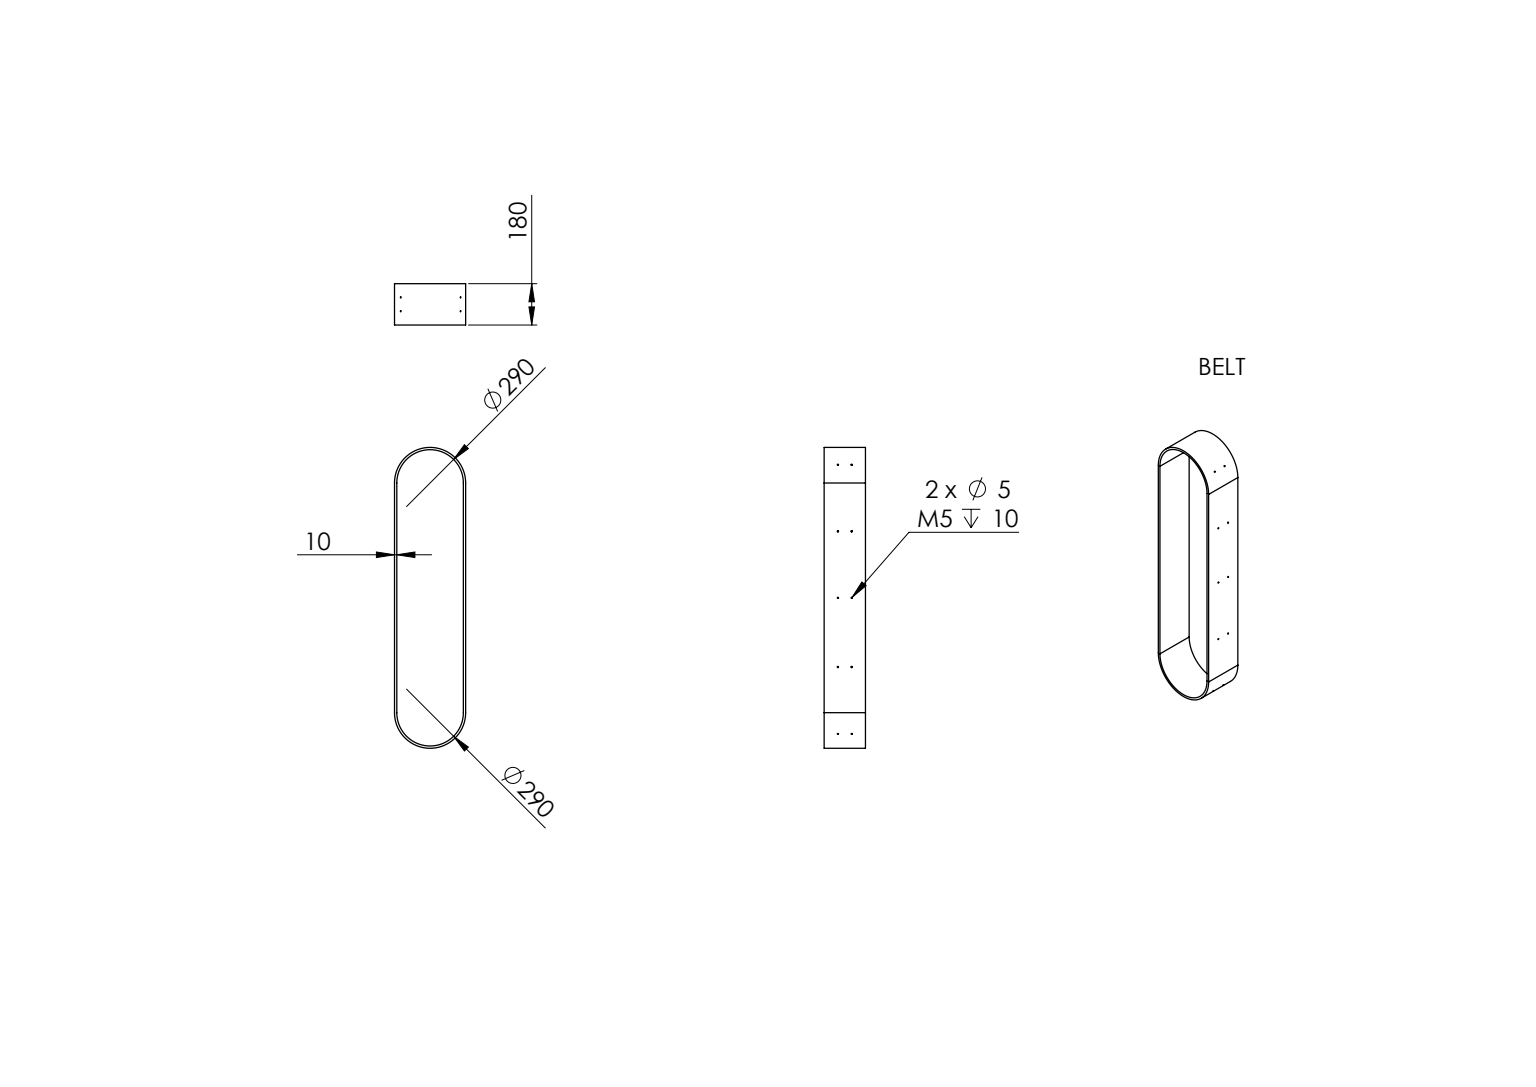
ISO-10303-21;
HEADER;
FILE_DESCRIPTION (('STEP AP214'),
    '1' );
FILE_NAME ('belt.step',
    '2026-10-31T03:46:07',
    ( '' ),
    ( '' ),
    'SwSTEP 2.0',
    'SolidWorks 2026',
    '' );
FILE_SCHEMA (( 'AUTOMOTIVE_DESIGN' ));
ENDSEC;

DATA;
#1=DIRECTION ( 'NONE',  ( -0.000000000000000000, -0.000000000000000000, -1.000000000000000000 ) ) ;
#9=CARTESIAN_POINT ( 'NONE',  ( 155.0000000000000568, -1000.000000000000000, 90.00000000000000000 ) ) ;
#15=AXIS2_PLACEMENT_3D ( 'NONE', #6057, #12994, #3756 ) ;
#18=CIRCLE ( 'NONE', #21621, 2.499999999999998668 ) ;
#25=CARTESIAN_POINT ( 'NONE',  ( -128.2695163047654319, 87.01699568756248482, -27.57873596473009670 ) ) ;
#36=CARTESIAN_POINT ( 'NONE',  ( -146.0000000000001137, -204.4690652294807478, 27.94500000000641649 ) ) ;
#37=LINE ( 'NONE', #254, #11884 ) ;
#45=VERTEX_POINT ( 'NONE', #9 ) ;
#55=DIRECTION ( 'NONE',  ( 0.9289202219288174023, 0.3702799228849934510, 6.982962677686266711E-15 ) ) ;
#56=CARTESIAN_POINT ( 'NONE',  ( 133.4872637682705090, 78.77924338079024835, 32.17229779615544771 ) ) ;
#74=CARTESIAN_POINT ( 'NONE',  ( 126.3653543294811499, 77.28387428943223370, 30.00000000000641620 ) ) ;
#82=LINE ( 'NONE', #14822, #8863 ) ;
#83=FACE_OUTER_BOUND ( 'NONE', #5048, .T. ) ;
#104=DIRECTION ( 'NONE',  ( 0.4924295582441756136, -0.5074575156280946020, -0.7071067811865532349 ) ) ;
#107=EDGE_CURVE ( 'NONE', #20023, #9785, #19883, .T. ) ;
#111=CARTESIAN_POINT ( 'NONE',  ( -127.8094121079449081, 87.69139705313254751, -27.49999999999350919 ) ) ;
#113=CYLINDRICAL_SURFACE ( 'NONE', #13258, 2.500000000000002220 ) ;
#120=LINE ( 'NONE', #7470, #18771 ) ;
#144=CARTESIAN_POINT ( 'NONE',  ( -136.7455495141632014, -1072.977142426286946, -31.53250949154617189 ) ) ;
#149=EDGE_CURVE ( 'NONE', #7198, #16229, #4462, .T. ) ;
#150=CARTESIAN_POINT ( 'NONE',  ( -134.5566256099404825, -1076.938388239963842, 30.33200430454444785 ) ) ;
#153=ADVANCED_FACE ( 'NONE', ( #23660 ), #11773, .F. ) ;
#159=CARTESIAN_POINT ( 'NONE',  ( 125.5946212300931251, -1090.835042168281007, 31.66065886938999796 ) ) ;
#161=CARTESIAN_POINT ( 'NONE',  ( -129.3084827928275899, 85.46529914716332144, 30.33200430454444785 ) ) ;
#166=FACE_OUTER_BOUND ( 'NONE', #524, .T. ) ;
#170=B_SPLINE_CURVE_WITH_KNOTS ( 'NONE', 3,
 ( #22399, #16491, #3559, #1745, #10973, #23729, #1990, #12913, #5622, #7185, #14575, #13162, #16380, #9267, #21916, #7319, #18537, #13033, #1867, #10867, #14821, #16628, #20334, #18294, #9136, #12812, #18638, #15068, #11086, #11248, #14938, #14705 ),
 .UNSPECIFIED., .F., .F.,
 ( 4, 2, 2, 2, 2, 2, 2, 2, 2, 2, 2, 2, 2, 2, 2, 4 ),
 ( 1.551583845779545699E-17, 0.0004914281572964048763, 0.0009828563145927943570, 0.001474284471889183512, 0.001965712629185573102, 0.002457140786481962474, 0.002948568943778351412, 0.003931425258371110641, 0.004422853415667485702, 0.004914281572963859895, 0.005405709730260234956, 0.005897137887556608282, 0.006388566044852983343, 0.006879994202149357536, 0.007371422359445732597, 0.007862850516742106791 ),
 .UNSPECIFIED. ) ;
#173=CARTESIAN_POINT ( 'NONE',  ( 131.5154891841473841, 82.02850787876496952, -30.32849798811265885 ) ) ;
#178=AXIS2_PLACEMENT_3D ( 'NONE', #20566, #18993, #2455 ) ;
#181=AXIS2_PLACEMENT_3D ( 'NONE', #11379, #9543, #20890 ) ;
#184=DIRECTION ( 'NONE',  ( 0.000000000000000000, -1.000000000000000000, 0.000000000000000000 ) ) ;
#189=DIRECTION ( 'NONE',  ( 0.9289202219288174023, 0.3702799228849934510, 6.982962677686266711E-15 ) ) ;
#190=ORIENTED_EDGE ( 'NONE', *, *, #703, .F. ) ;
#192=DIRECTION ( 'NONE',  ( -0.9289202219288174023, -0.3702799228849933955, -6.982962677686267499E-15 ) ) ;
#204=CARTESIAN_POINT ( 'NONE',  ( 194.7499999999997442, -209.9999999999996874, 30.00000000000675726 ) ) ;
#208=DIRECTION ( 'NONE',  ( -1.350636282998972974E-14, 0.000000000000000000, -1.000000000000000000 ) ) ;
#221=CARTESIAN_POINT ( 'NONE',  ( -135.9481979339306577, -1074.452087582500553, 27.51597717546056643 ) ) ;
#223=VERTEX_POINT ( 'NONE', #18684 ) ;
#242=ORIENTED_EDGE ( 'NONE', *, *, #6175, .T. ) ;
#250=DIRECTION ( 'NONE',  ( -0.000000000000000000, -0.000000000000000000, -1.000000000000000000 ) ) ;
#254=CARTESIAN_POINT ( 'NONE',  ( 194.7500000000001705, -210.0000000000003411, -27.49999999999322498 ) ) ;
#274=ORIENTED_EDGE ( 'NONE', *, *, #4252, .F. ) ;
#275=CARTESIAN_POINT ( 'NONE',  ( 125.1337793500219817, -1091.468903702553689, 27.75096515221187232 ) ) ;
#277=AXIS2_PLACEMENT_3D ( 'NONE', #7099, #10883, #12700 ) ;
#278=CARTESIAN_POINT ( 'NONE',  ( -127.9949300873395543, 87.42039156790949050, 32.50000000000647304 ) ) ;
#279=EDGE_CURVE ( 'NONE', #7198, #16055, #16896, .T. ) ;
#283=ORIENTED_EDGE ( 'NONE', *, *, #21682, .F. ) ;
#288=EDGE_CURVE ( 'NONE', #16653, #6623, #20746, .T. ) ;
#290=CARTESIAN_POINT ( 'NONE',  ( 132.6714475832646656, 80.14557597090949059, -27.51562286569268423 ) ) ;
#295=VECTOR ( 'NONE', #20136, 1000.000000000000000 ) ;
#299=ORIENTED_EDGE ( 'NONE', *, *, #12045, .F. ) ;
#314=AXIS2_PLACEMENT_3D ( 'NONE', #11031, #20164, #12506 ) ;
#323=CYLINDRICAL_SURFACE ( 'NONE', #9568, 2.500000000000002220 ) ;
#349=ORIENTED_EDGE ( 'NONE', *, *, #18259, .F. ) ;
#360=AXIS2_PLACEMENT_3D ( 'NONE', #12995, #16243, #18159 ) ;
#361=CIRCLE ( 'NONE', #6148, 2.055000000000001492 ) ;
#365=CARTESIAN_POINT ( 'NONE',  ( -127.2680799365782889, 88.47518962644093676, 27.75040112528346015 ) ) ;
#371=AXIS2_PLACEMENT_3D ( 'NONE', #23355, #14098, #23119 ) ;
#378=EDGE_LOOP ( 'NONE', ( #19734, #5802 ) ) ;
#380=VECTOR ( 'NONE', #18750, 1000.000000000000114 ) ;
#392=ORIENTED_EDGE ( 'NONE', *, *, #11920, .F. ) ;
#394=AXIS2_PLACEMENT_3D ( 'NONE', #13322, #2647, #11500 ) ;
#401=CARTESIAN_POINT ( 'NONE',  ( -135.6291186032800340, -1075.032345129804526, 27.50000000000644462 ) ) ;
#404=VERTEX_POINT ( 'NONE', #6272 ) ;
#412=CARTESIAN_POINT ( 'NONE',  ( -128.8385278530645905, 86.17219694792730422, 28.11255663403418126 ) ) ;
#415=EDGE_CURVE ( 'NONE', #12774, #3203, #17606, .T. ) ;
#420=ORIENTED_EDGE ( 'NONE', *, *, #2725, .F. ) ;
#426=CARTESIAN_POINT ( 'NONE',  ( 132.5032837044622056, 80.42329363488276783, -27.57873596473011446 ) ) ;
#439=DIRECTION ( 'NONE',  ( 1.000000000000000000, -0.000000000000000000, 6.982962677686266711E-15 ) ) ;
#455=ORIENTED_EDGE ( 'NONE', *, *, #19160, .F. ) ;
#457=CARTESIAN_POINT ( 'NONE',  ( 153.5653415408403646, -1122.352966361445169, 30.00000000000675726 ) ) ;
#462=DIRECTION ( 'NONE',  ( -0.7232617928448825673, 0.6905739489807055653, 6.982962677686266711E-15 ) ) ;
#471=VERTEX_POINT ( 'NONE', #10993 ) ;
#480=CARTESIAN_POINT ( 'NONE',  ( -146.4450000000005332, -784.4690652294799520, -29.99999999999356248 ) ) ;
#483=CARTESIAN_POINT ( 'NONE',  ( -127.9021285790841205, 87.55595642181887683, 27.50000000000646239 ) ) ;
#493=VERTEX_POINT ( 'NONE', #1420 ) ;
#507=CARTESIAN_POINT ( 'NONE',  ( -136.9304241666588666, -1072.629629052829387, -29.19154146838981490 ) ) ;
#512=ORIENTED_EDGE ( 'NONE', *, *, #2203, .T. ) ;
#513=DIRECTION ( 'NONE',  ( -0.7071067811865320296, 9.875400524328840493E-15, 0.7071067811865631159 ) ) ;
#524=EDGE_LOOP ( 'NONE', ( #4189, #16667, #22630, #21113 ) ) ;
#547=ORIENTED_EDGE ( 'NONE', *, *, #19326, .F. ) ;
#572=ORIENTED_EDGE ( 'NONE', *, *, #16103, .T. ) ;
#586=CARTESIAN_POINT ( 'NONE',  ( -146.0000000000005684, -496.5240652294801293, -29.99999999999356604 ) ) ;
#590=VERTEX_POINT ( 'NONE', #22650 ) ;
#597=DIRECTION ( 'NONE',  ( 1.000000000000000000, -0.000000000000000000, 6.982962677686266711E-15 ) ) ;
#598=CARTESIAN_POINT ( 'NONE',  ( -126.4561707720357191, 89.63167338449062527, 29.67072815018523357 ) ) ;
#619=EDGE_CURVE ( 'NONE', #20328, #13113, #6356, .T. ) ;
#624=CARTESIAN_POINT ( 'NONE',  ( -136.9597779064870053, -1072.574344195403910, -30.66034227022094072 ) ) ;
#634=DIRECTION ( 'NONE',  ( -1.000000000000000000, 1.408839003528726857E-14, 6.982962677686266711E-15 ) ) ;
#648=CARTESIAN_POINT ( 'NONE',  ( 155.0000000000000568, -801.0618695410399823, 32.50000000000648015 ) ) ;
#656=DIRECTION ( 'NONE',  ( 1.350636282998972974E-14, 0.000000000000000000, -1.000000000000000000 ) ) ;
#658=ORIENTED_EDGE ( 'NONE', *, *, #12364, .F. ) ;
#667=VECTOR ( 'NONE', #14846, 1000.000000000000114 ) ;
#676=VECTOR ( 'NONE', #16342, 1000.000000000000000 ) ;
#677=DIRECTION ( 'NONE',  ( 1.350636282998972974E-14, 0.000000000000000000, -1.000000000000000000 ) ) ;
#703=EDGE_CURVE ( 'NONE', #23044, #590, #11400, .T. ) ;
#706=EDGE_CURVE ( 'NONE', #3521, #2188, #19499, .T. ) ;
#716=ORIENTED_EDGE ( 'NONE', *, *, #17409, .T. ) ;
#717=ORIENTED_EDGE ( 'NONE', *, *, #4723, .F. ) ;
#726=DIRECTION ( 'NONE',  ( 1.000000000000000000, -0.000000000000000000, 6.982962677686266711E-15 ) ) ;
#732=DIRECTION ( 'NONE',  ( -0.000000000000000000, 0.000000000000000000, -1.000000000000000000 ) ) ;
#742=ADVANCED_FACE ( 'NONE', ( #13655 ), #12191, .F. ) ;
#750=CARTESIAN_POINT ( 'NONE',  ( -127.9021285790841205, 87.55595642181886262, 32.50000000000646594 ) ) ;
#782=CIRCLE ( 'NONE', #20051, 2.499999999999998668 ) ;
#784=VERTEX_POINT ( 'NONE', #15907 ) ;
#790=EDGE_CURVE ( 'NONE', #2904, #12317, #6354, .T. ) ;
#794=CARTESIAN_POINT ( 'NONE',  ( -135.7895026000616951, -1074.740959209979792, -32.49999999999351985 ) ) ;
#800=ORIENTED_EDGE ( 'NONE', *, *, #9748, .T. ) ;
#802=DIRECTION ( 'NONE',  ( -1.350636282998972974E-14, 0.000000000000000000, -1.000000000000000000 ) ) ;
#803=DIRECTION ( 'NONE',  ( 1.110223024625157172E-14, 0.000000000000000000, -1.000000000000000000 ) ) ;
#816=ADVANCED_FACE ( 'NONE', ( #4674 ), #21087, .F. ) ;
#825=EDGE_LOOP ( 'NONE', ( #14289, #18811, #20424, #21702 ) ) ;
#828=DIRECTION ( 'NONE',  ( 0.000000000000000000, 0.000000000000000000, -1.000000000000000000 ) ) ;
#834=CARTESIAN_POINT ( 'NONE',  ( -134.7167544493340472, -1076.657711551589273, -28.73951976925632223 ) ) ;
#846=VERTEX_POINT ( 'NONE', #23494 ) ;
#854=ORIENTED_EDGE ( 'NONE', *, *, #6766, .T. ) ;
#860=ORIENTED_EDGE ( 'NONE', *, *, #4723, .T. ) ;
#871=EDGE_CURVE ( 'NONE', #8499, #16240, #17927, .T. ) ;
#885=VERTEX_POINT ( 'NONE', #4487 ) ;
#886=FACE_OUTER_BOUND ( 'NONE', #15033, .T. ) ;
#900=DIRECTION ( 'NONE',  ( 0.7071067811865320296, 8.659560562355062281E-17, 0.7071067811865631159 ) ) ;
#902=FACE_OUTER_BOUND ( 'NONE', #12806, .T. ) ;
#907=VERTEX_POINT ( 'NONE', #17295 ) ;
#910=CARTESIAN_POINT ( 'NONE',  ( 145.0000000000000284, 0.000000000000000000, -90.00000000000000000 ) ) ;
#911=ADVANCED_FACE ( 'NONE', ( #9367 ), #17415, .F. ) ;
#924=DIRECTION ( 'NONE',  ( -1.000000000000000000, 1.408839003528726857E-14, 6.982962677686266711E-15 ) ) ;
#927=CARTESIAN_POINT ( 'NONE',  ( -146.0000000000000568, -784.4690652294805204, 32.05500000000641592 ) ) ;
#941=CARTESIAN_POINT ( 'NONE',  ( -127.9021285790841205, 87.55595642181886262, 32.50000000000646594 ) ) ;
#942=CIRCLE ( 'NONE', #6346, 2.500000000000002220 ) ;
#944=CARTESIAN_POINT ( 'NONE',  ( -135.2464651929980164, -1075.719328653694674, -32.24903484778816676 ) ) ;
#946=CONICAL_SURFACE ( 'NONE', #22543, 2.055000000000001492, 0.7853981633974633780 ) ;
#950=ORIENTED_EDGE ( 'NONE', *, *, #15583, .F. ) ;
#951=CARTESIAN_POINT ( 'NONE',  ( 133.6256533058505340, 78.54427823740819292, -31.99339931332764664 ) ) ;
#963=VERTEX_POINT ( 'NONE', #1980 ) ;
#970=AXIS2_PLACEMENT_3D ( 'NONE', #14005, #15567, #10496 ) ;
#979=ORIENTED_EDGE ( 'NONE', *, *, #3400, .T. ) ;
#984=EDGE_LOOP ( 'NONE', ( #10266, #7109, #23635, #16321 ) ) ;
#992=CARTESIAN_POINT ( 'NONE',  ( -155.0000000000000284, -784.4690652294804067, 30.00000000000648015 ) ) ;
#998=FACE_OUTER_BOUND ( 'NONE', #17064, .T. ) ;
#1013=DIRECTION ( 'NONE',  ( -0.7232617928448825673, 0.6905739489807055653, 6.982962677686266711E-15 ) ) ;
#1014=ORIENTED_EDGE ( 'NONE', *, *, #14681, .T. ) ;
#1026=CARTESIAN_POINT ( 'NONE',  ( 132.1831532210145781, 80.94878845338391216, 32.18904844917290831 ) ) ;
#1028=EDGE_CURVE ( 'NONE', #3982, #8260, #19323, .T. ) ;
#1034=CARTESIAN_POINT ( 'NONE',  ( 145.9999999999997726, -209.9999999999996874, 32.05500000000641592 ) ) ;
#1052=B_SPLINE_CURVE_WITH_KNOTS ( 'NONE', 3,
 ( #9232, #278, #22370, #3531, #9350, #10941, #2076, #20438, #7635, #13244, #13126, #18510, #14673, #161, #12780, #11057, #16464, #1716, #20548, #1964, #7407, #412, #3999, #11418, #15149, #2190, #14906, #9583 ),
 .UNSPECIFIED., .F., .F.,
 ( 4, 2, 2, 2, 2, 2, 2, 2, 2, 2, 2, 2, 2, 4 ),
 ( 0.007862850516742138016, 0.008354729399060728881, 0.008846608281379319746, 0.009830366046016465048, 0.01032224492833501775, 0.01081412381065357219, 0.01130600269297213530, 0.01179788157529069667, 0.01278163933992781248, 0.01327351822224636518, 0.01376539710456491789, 0.01425727598688347232, 0.01474915486920202502, 0.01573291263383913910 ),
 .UNSPECIFIED. ) ;
#1060=DIRECTION ( 'NONE',  ( 6.982962677686266711E-15, -9.837870180509810443E-29, 1.000000000000000000 ) ) ;
#1066=ORIENTED_EDGE ( 'NONE', *, *, #17131, .T. ) ;
#1070=EDGE_LOOP ( 'NONE', ( #5859, #20179, #7990, #3213 ) ) ;
#1071=CARTESIAN_POINT ( 'NONE',  ( 134.1261853992453723, 77.68633335585815303, -30.32927184981474866 ) ) ;
#1074=EDGE_CURVE ( 'NONE', #19239, #3203, #19111, .T. ) ;
#1078=DIRECTION ( 'NONE',  ( 0.000000000000000000, 0.000000000000000000, -1.000000000000000000 ) ) ;
#1086=ORIENTED_EDGE ( 'NONE', *, *, #14681, .F. ) ;
#1095=AXIS2_PLACEMENT_3D ( 'NONE', #9625, #16992, #2360 ) ;
#1107=DIRECTION ( 'NONE',  ( 1.000000000000000000, -0.000000000000000000, 6.982962677686266711E-15 ) ) ;
#1168=LINE ( 'NONE', #10860, #8480 ) ;
#1195=EDGE_CURVE ( 'NONE', #19464, #19646, #9096, .T. ) ;
#1205=CARTESIAN_POINT ( 'NONE',  ( 133.2566323304059495, 79.16876461166333456, -32.37389708099360774 ) ) ;
#1223=CARTESIAN_POINT ( 'NONE',  ( -136.9835704417550915, -1072.529321614197215, 30.32918505548582644 ) ) ;
#1231=DIRECTION ( 'NONE',  ( -0.9423651898111408132, -0.3345860861306287348, 6.982962677686266711E-15 ) ) ;
#1233=ORIENTED_EDGE ( 'NONE', *, *, #18027, .F. ) ;
#1248=CARTESIAN_POINT ( 'NONE',  ( 145.9999999999998010, -207.9449999999996805, 30.00000000000641620 ) ) ;
#1252=AXIS2_PLACEMENT_3D ( 'NONE', #4431, #462, #11840 ) ;
#1255=CARTESIAN_POINT ( 'NONE',  ( 155.0000000000000284, 2.775557561562891351E-16, 90.00000000000000000 ) ) ;
#1258=LINE ( 'NONE', #23228, #15953 ) ;
#1268=VERTEX_POINT ( 'NONE', #5671 ) ;
#1271=LINE ( 'NONE', #910, #18058 ) ;
#1282=ORIENTED_EDGE ( 'NONE', *, *, #18033, .T. ) ;
#1296=VECTOR ( 'NONE', #8454, 1000.000000000000000 ) ;
#1299=CIRCLE ( 'NONE', #4783, 2.499999999999998668 ) ;
#1304=FACE_OUTER_BOUND ( 'NONE', #3498, .T. ) ;
#1362=ORIENTED_EDGE ( 'NONE', *, *, #22126, .F. ) ;
#1367=VECTOR ( 'NONE', #17921, 1000.000000000000000 ) ;
#1372=EDGE_LOOP ( 'NONE', ( #10743, #20653, #3624, #2809 ) ) ;
#1373=CARTESIAN_POINT ( 'NONE',  ( 133.9567665909156915, 77.97815834559359871, 31.25900233431400110 ) ) ;
#1387=AXIS2_PLACEMENT_3D ( 'NONE', #13984, #21307, #4758 ) ;
#1393=VECTOR ( 'NONE', #20319, 1000.000000000000000 ) ;
#1395=DIRECTION ( 'NONE',  ( 1.000000000000000000, -0.000000000000000000, -0.000000000000000000 ) ) ;
#1396=EDGE_LOOP ( 'NONE', ( #13575, #10334, #6051, #16215 ) ) ;
#1405=LINE ( 'NONE', #21806, #15791 ) ;
#1411=ORIENTED_EDGE ( 'NONE', *, *, #22522, .F. ) ;
#1420=CARTESIAN_POINT ( 'NONE',  ( 155.0000000000000284, 2.775557561562891351E-16, 90.00000000000000000 ) ) ;
#1423=FACE_OUTER_BOUND ( 'NONE', #3117, .T. ) ;
#1434=CARTESIAN_POINT ( 'NONE',  ( -145.0000000000000284, -1000.000000000000000, 90.00000000000000000 ) ) ;
#1440=AXIS2_PLACEMENT_3D ( 'NONE', #204, #3567, #20000 ) ;
#1441=ORIENTED_EDGE ( 'NONE', *, *, #20361, .T. ) ;
#1457=DIRECTION ( 'NONE',  ( 1.000000000000000000, 0.000000000000000000, -0.000000000000000000 ) ) ;
#1459=AXIS2_PLACEMENT_3D ( 'NONE', #457, #15441, #6245 ) ;
#1463=SHAPE_REPRESENTATION_RELATIONSHIP ( 'NONE' , 'NONE' ,  #4684, #5256 ) ;
#1478=AXIS2_PLACEMENT_3D ( 'NONE', #9714, #10185, #9952 ) ;
#1479=EDGE_CURVE ( 'NONE', #8566, #22288, #7241, .T. ) ;
#1495=CIRCLE ( 'NONE', #1095, 2.499999999999998668 ) ;
#1503=DIRECTION ( 'NONE',  ( -6.486615240276975916E-15, -2.585650881802458380E-15, 1.000000000000000000 ) ) ;
#1512=EDGE_CURVE ( 'NONE', #16414, #21068, #17546, .T. ) ;
#1520=ORIENTED_EDGE ( 'NONE', *, *, #21180, .F. ) ;
#1542=STYLED_ITEM ( 'NONE', ( #11425 ), #5256 ) ;
#1546=AXIS2_PLACEMENT_3D ( 'NONE', #9149, #17967, #22161 ) ;
#1556=ORIENTED_EDGE ( 'NONE', *, *, #12045, .T. ) ;
#1560=CARTESIAN_POINT ( 'NONE',  ( 126.3653543294818178, 77.28387428943173632, -32.05499999999358351 ) ) ;
#1561=CONICAL_SURFACE ( 'NONE', #10003, 2.055000000000001492, 0.7853981633974633780 ) ;
#1562=EDGE_LOOP ( 'NONE', ( #23282, #1362, #17315, #5755 ) ) ;
#1580=ORIENTED_EDGE ( 'NONE', *, *, #6702, .T. ) ;
#1588=CARTESIAN_POINT ( 'NONE',  ( 124.6683470056595127, -1092.102735484117147, -32.49999999999354117 ) ) ;
#1591=CARTESIAN_POINT ( 'NONE',  ( 145.0000000000000284, 0.000000000000000000, 90.00000000000000000 ) ) ;
#1602=ADVANCED_FACE ( 'NONE', ( #1423 ), #18316, .F. ) ;
#1608=CARTESIAN_POINT ( 'NONE',  ( 124.4701338314437891, -1092.369831568442805, 27.50000000000646239 ) ) ;
#1612=CARTESIAN_POINT ( 'NONE',  ( 133.1760469597742542, 79.30426557766963924, 32.42079297023035167 ) ) ;
#1633=EDGE_CURVE ( 'NONE', #7326, #9978, #7511, .T. ) ;
#1671=CARTESIAN_POINT ( 'NONE',  ( -126.4656051290183285, 89.61836744852109859, -29.67081494451417001 ) ) ;
#1672=PLANE ( 'NONE',  #9200 ) ;
#1685=VECTOR ( 'NONE', #19508, 1000.000000000000000 ) ;
#1686=VERTEX_POINT ( 'NONE', #6000 ) ;
#1688=AXIS2_PLACEMENT_3D ( 'NONE', #10735, #16493, #17957 ) ;
#1690=EDGE_LOOP ( 'NONE', ( #6686, #8215, #23216, #20846 ) ) ;
#1692=CARTESIAN_POINT ( 'NONE',  ( -124.2796999450275450, 81.25594874576316329, -29.99999999999356604 ) ) ;
#1695=EDGE_LOOP ( 'NONE', ( #19166, #21461, #15410, #19396 ) ) ;
#1698=AXIS2_PLACEMENT_3D ( 'NONE', #7708, #22425, #5886 ) ;
#1704=DIRECTION ( 'NONE',  ( 0.000000000000000000, 0.000000000000000000, -1.000000000000000000 ) ) ;
#1706=FACE_OUTER_BOUND ( 'NONE', #17410, .T. ) ;
#1712=ORIENTED_EDGE ( 'NONE', *, *, #6318, .T. ) ;
#1715=VERTEX_POINT ( 'NONE', #9760 ) ;
#1716=CARTESIAN_POINT ( 'NONE',  ( -129.1746529357998270, 85.66745698985749868, 28.88700448195642068 ) ) ;
#1722=DIRECTION ( 'NONE',  ( 0.6568457881071740889, 0.2618274444092085762, -0.7071067811865532349 ) ) ;
#1729=EDGE_CURVE ( 'NONE', #14202, #15482, #20862, .T. ) ;
#1731=LINE ( 'NONE', #7301, #9257 ) ;
#1735=CLOSED_SHELL ( 'NONE', ( #13363, #16071, #9628, #22127, #8705, #21441, #8757, #1602, #22748, #9080, #14947, #13025, #14476, #19578, #2546, #7223, #10942, #8896, #15552, #7130, #7059, #20518, #17509, #23348, #23768, #9961, #14916, #18560, #153, #2149, #3503, #816, #18070, #11756, #10182, #7282, #6829, #11757, #23281, #7968, #2240, #22742, #18986, #7336, #15830, #911, #9920, #22834, #16286, #22037, #12930, #23177, #7926, #19756, #3416, #16865, #6167, #17306, #11112, #15935, #9576, #16560, #742, #10355, #5623, #4008, #17245, #9140, #5438, #18901, #2071, #16252, #20434, #12891, #9756, #17939, #8043, #12470, #15163, #17696, #12959, #9190, #8118, #16640, #23620, #18287, #16603, #2687, #21080, #8934, #2478, #18885, #21715, #6232, #3886, #7532, #2388, #10074, #11374, #13764, #18244, #4455, #21245, #5079 ) ) ;
#1745=CARTESIAN_POINT ( 'NONE',  ( 124.0809974055272704, -1092.892044598690291, -32.42132972170173133 ) ) ;
#1774=CARTESIAN_POINT ( 'NONE',  ( -135.8696211158498386, -1074.595399753385209, 27.50000000000646949 ) ) ;
#1786=LINE ( 'NONE', #12951, #18991 ) ;
#1787=ORIENTED_EDGE ( 'NONE', *, *, #4137, .F. ) ;
#1790=CIRCLE ( 'NONE', #9160, 2.500000000000002220 ) ;
#1815=AXIS2_PLACEMENT_3D ( 'NONE', #8788, #21805, #10733 ) ;
#1817=EDGE_LOOP ( 'NONE', ( #14714, #23618 ) ) ;
#1826=AXIS2_PLACEMENT_3D ( 'NONE', #9456, #16809, #18720 ) ;
#1835=CARTESIAN_POINT ( 'NONE',  ( 133.2566323304055800, 79.16876461166395984, 27.62610291900640291 ) ) ;
#1851=DIRECTION ( 'NONE',  ( -1.000000000000000000, 0.000000000000000000, 0.000000000000000000 ) ) ;
#1857=EDGE_CURVE ( 'NONE', #8155, #19239, #16024, .T. ) ;
#1862=EDGE_CURVE ( 'NONE', #23140, #13840, #11917, .T. ) ;
#1867=CARTESIAN_POINT ( 'NONE',  ( 123.0250976530550133, -1094.285891978964401, -29.19154146838977226 ) ) ;
#1868=CARTESIAN_POINT ( 'NONE',  ( -155.0000000000000284, -1000.000000000000000, -90.00000000000000000 ) ) ;
#1882=AXIS2_PLACEMENT_3D ( 'NONE', #10560, #10088, #17428 ) ;
#1898=ORIENTED_EDGE ( 'NONE', *, *, #3129, .T. ) ;
#1899=ORIENTED_EDGE ( 'NONE', *, *, #8577, .F. ) ;
#1928=VERTEX_POINT ( 'NONE', #16265 ) ;
#1931=ORIENTED_EDGE ( 'NONE', *, *, #14365, .T. ) ;
#1937=CARTESIAN_POINT ( 'NONE',  ( 125.4586218058184670, -1091.022788359629203, -31.88744336596587559 ) ) ;
#1941=EDGE_CURVE ( 'NONE', #17109, #11264, #3550, .T. ) ;
#1945=ORIENTED_EDGE ( 'NONE', *, *, #21631, .F. ) ;
#1946=EDGE_CURVE ( 'NONE', #493, #784, #2228, .T. ) ;
#1949=CARTESIAN_POINT ( 'NONE',  ( -135.8686487629348676, -1074.597166325825583, -27.49999999999351985 ) ) ;
#1953=CARTESIAN_POINT ( 'NONE',  ( -134.6139742523213272, -1076.838024977515715, 30.81384172145502731 ) ) ;
#1964=CARTESIAN_POINT ( 'NONE',  ( -129.0286178947084466, 85.88727694560715520, 28.47118012353584859 ) ) ;
#1976=ORIENTED_EDGE ( 'NONE', *, *, #4096, .F. ) ;
#1978=CARTESIAN_POINT ( 'NONE',  ( 155.0000000000000284, -500.0000000000000000, -32.49999999999997158 ) ) ;
#1980=CARTESIAN_POINT ( 'NONE',  ( 155.0000000000000284, -500.0000000000000000, 27.50000000000001066 ) ) ;
#1986=DIRECTION ( 'NONE',  ( 1.350636282998972974E-14, 0.000000000000000000, -1.000000000000000000 ) ) ;
#1990=CARTESIAN_POINT ( 'NONE',  ( 123.7141469857648559, -1093.380023028672440, -32.17346063704734860 ) ) ;
#1993=DIRECTION ( 'NONE',  ( -0.5114233182937452105, 0.4883095222350190001, 0.7071067811865631159 ) ) ;
#2003=FACE_OUTER_BOUND ( 'NONE', #15550, .T. ) ;
#2005=DIRECTION ( 'NONE',  ( -1.000000000000000000, -2.775557561562891351E-17, 0.000000000000000000 ) ) ;
#2010=ORIENTED_EDGE ( 'NONE', *, *, #19334, .T. ) ;
#2012=CARTESIAN_POINT ( 'NONE',  ( -136.6960319176257883, -1073.069888270695401, 28.34183984639752651 ) ) ;
#2037=VERTEX_POINT ( 'NONE', #10722 ) ;
#2054=CARTESIAN_POINT ( 'NONE',  ( -136.5237489982507100, -1073.391313005787424, -31.99339931332765374 ) ) ;
#2071=ADVANCED_FACE ( 'NONE', ( #7655 ), #15697, .F. ) ;
#2076=CARTESIAN_POINT ( 'NONE',  ( -128.7717867965311598, 86.27213916325780474, 32.00444854364504010 ) ) ;
#2079=CIRCLE ( 'NONE', #5950, 2.500000000000002220 ) ;
#2091=AXIS2_PLACEMENT_3D ( 'NONE', #15406, #19116, #6576 ) ;
#2093=DIRECTION ( 'NONE',  ( -1.110223024625155594E-14, 0.000000000000000000, -1.000000000000000000 ) ) ;
#2115=DIRECTION ( 'NONE',  ( 1.000000000000000000, -0.000000000000000000, 6.982962677686266711E-15 ) ) ;
#2126=LINE ( 'NONE', #5879, #22069 ) ;
#2127=CARTESIAN_POINT ( 'NONE',  ( 146.0000000000001990, -210.0000000000003411, -27.94499999999356632 ) ) ;
#2137=CARTESIAN_POINT ( 'NONE',  ( -146.4450000000000784, -204.4690652294807194, 30.00000000000641975 ) ) ;
#2149=ADVANCED_FACE ( 'NONE', ( #9603 ), #11320, .F. ) ;
#2156=CARTESIAN_POINT ( 'NONE',  ( -129.0286178947080771, 85.88727694560768100, -31.52881987646414430 ) ) ;
#2174=AXIS2_PLACEMENT_3D ( 'NONE', #15138, #20655, #4110 ) ;
#2177=CARTESIAN_POINT ( 'NONE',  ( -134.8603954219443608, -1076.404761192049591, 28.34264858295328438 ) ) ;
#2188=VERTEX_POINT ( 'NONE', #20687 ) ;
#2190=CARTESIAN_POINT ( 'NONE',  ( -128.2758413234849399, 87.00805048166478173, 27.56549073392523397 ) ) ;
#2196=EDGE_CURVE ( 'NONE', #14422, #19693, #11391, .T. ) ;
#2203=EDGE_CURVE ( 'NONE', #13113, #20328, #942, .T. ) ;
#2205=DIRECTION ( 'NONE',  ( -0.000000000000000000, -0.000000000000000000, -1.000000000000000000 ) ) ;
#2212=CARTESIAN_POINT ( 'NONE',  ( 123.9854850298566618, -1093.019475613609529, 32.37408494914630808 ) ) ;
#2223=CARTESIAN_POINT ( 'NONE',  ( -155.0000000000000284, 0.000000000000000000, -90.00000000000000000 ) ) ;
#2228=CIRCLE ( 'NONE', #5325, 155.0000000000000284 ) ;
#2229=DIRECTION ( 'NONE',  ( 1.110223024625155594E-14, 0.000000000000000000, -1.000000000000000000 ) ) ;
#2235=FACE_OUTER_BOUND ( 'NONE', #21609, .T. ) ;
#2240=ADVANCED_FACE ( 'NONE', ( #998, #21301 ), #13978, .F. ) ;
#2243=CIRCLE ( 'NONE', #5404, 2.500000000000002220 ) ;
#2267=DIRECTION ( 'NONE',  ( 1.350636282998972974E-14, 0.000000000000000000, -1.000000000000000000 ) ) ;
#2271=PRODUCT_DEFINITION_CONTEXT ( 'detailed design', #7866, 'design' ) ;
#2273=ORIENTED_EDGE ( 'NONE', *, *, #5882, .T. ) ;
#2294=CARTESIAN_POINT ( 'NONE',  ( 145.9999999999998010, -209.9999999999996874, 30.00000000000641620 ) ) ;
#2306=AXIS2_PLACEMENT_3D ( 'NONE', #17479, #924, #6615 ) ;
#2307=CARTESIAN_POINT ( 'NONE',  ( -136.1024116720897723, -1074.169801158669088, -32.42132972170178107 ) ) ;
#2315=CIRCLE ( 'NONE', #14619, 2.499999999999998668 ) ;
#2329=ORIENTED_EDGE ( 'NONE', *, *, #19411, .T. ) ;
#2348=EDGE_CURVE ( 'NONE', #1928, #2426, #8066, .T. ) ;
#2360=DIRECTION ( 'NONE',  ( -1.110223024625157172E-14, 0.000000000000000000, -1.000000000000000000 ) ) ;
#2385=EDGE_LOOP ( 'NONE', ( #14988, #20099 ) ) ;
#2388=ADVANCED_FACE ( 'NONE', ( #6805 ), #16242, .F. ) ;
#2390=CARTESIAN_POINT ( 'NONE',  ( -123.1824219776882785, 83.04955713735500922, 32.50000000000641620 ) ) ;
#2399=EDGE_LOOP ( 'NONE', ( #14268, #6366, #3728, #21228 ) ) ;
#2403=DIRECTION ( 'NONE',  ( 0.6964005597823107463, -0.7176533009294141507, 6.982962677686266711E-15 ) ) ;
#2422=CARTESIAN_POINT ( 'NONE',  ( -136.3242110351077372, -1073.761323382753289, -27.75009929603931980 ) ) ;
#2424=EDGE_LOOP ( 'NONE', ( #2273, #11811 ) ) ;
#2425=CARTESIAN_POINT ( 'NONE',  ( -135.7895026000614109, -1074.740959209980247, 32.50000000000646594 ) ) ;
#2426=VERTEX_POINT ( 'NONE', #23690 ) ;
#2432=CYLINDRICAL_SURFACE ( 'NONE', #7672, 2.500000000000002220 ) ;
#2444=( LENGTH_UNIT ( ) NAMED_UNIT ( * ) SI_UNIT ( .MILLI., .METRE. ) );
#2455=DIRECTION ( 'NONE',  ( 0.000000000000000000, 0.000000000000000000, -1.000000000000000000 ) ) ;
#2457=CARTESIAN_POINT ( 'NONE',  ( 124.3723197571909793, -1092.501637924545321, 32.50000000000647304 ) ) ;
#2471=CARTESIAN_POINT ( 'NONE',  ( -155.0000000000000284, -204.4690652294799520, -32.49999999999350564 ) ) ;
#2478=ADVANCED_FACE ( 'NONE', ( #12417 ), #3168, .F. ) ;
#2485=ORIENTED_EDGE ( 'NONE', *, *, #3147, .T. ) ;
#2490=CIRCLE ( 'NONE', #9055, 2.499999999999998668 ) ;
#2504=DIRECTION ( 'NONE',  ( -1.350636282998972974E-14, 0.000000000000000000, -1.000000000000000000 ) ) ;
#2511=CARTESIAN_POINT ( 'NONE',  ( -122.8605704798722087, 82.74225173005940803, -32.05499999999356930 ) ) ;
#2519=PLANE ( 'NONE',  #19938 ) ;
#2521=EDGE_LOOP ( 'NONE', ( #15122, #7804, #420, #6250 ) ) ;
#2543=FACE_BOUND ( 'NONE', #378, .T. ) ;
#2546=ADVANCED_FACE ( 'NONE', ( #18847 ), #11188, .F. ) ;
#2561=ORIENTED_EDGE ( 'NONE', *, *, #9886, .T. ) ;
#2565=ORIENTED_EDGE ( 'NONE', *, *, #1074, .F. ) ;
#2567=CARTESIAN_POINT ( 'NONE',  ( -146.4450000000005332, -784.4690652294799520, -32.49999999999356248 ) ) ;
#2568=CARTESIAN_POINT ( 'NONE',  ( 132.0389103176324568, 81.18340533128207426, -31.99040335529153367 ) ) ;
#2586=ORIENTED_EDGE ( 'NONE', *, *, #22003, .F. ) ;
#2607=CARTESIAN_POINT ( 'NONE',  ( 131.5158088764650586, 82.02799531629221974, 30.16873261443286580 ) ) ;
#2622=CARTESIAN_POINT ( 'NONE',  ( -155.0000000000000284, -784.4690652294798383, -32.49999999999350564 ) ) ;
#2623=CARTESIAN_POINT ( 'NONE',  ( -146.4450000000005332, -494.4690652294800657, -29.99999999999356248 ) ) ;
#2625=ORIENTED_EDGE ( 'NONE', *, *, #10506, .F. ) ;
#2626=ORIENTED_EDGE ( 'NONE', *, *, #3852, .T. ) ;
#2628=DIRECTION ( 'NONE',  ( -0.9423651898111408132, -0.3345860861306287348, 6.982962677686266711E-15 ) ) ;
#2635=VECTOR ( 'NONE', #21326, 1000.000000000000000 ) ;
#2647=DIRECTION ( 'NONE',  ( 0.9289202219288174023, 0.3702799228849934510, 6.982962677686266711E-15 ) ) ;
#2652=CIRCLE ( 'NONE', #21166, 2.500000000000002220 ) ;
#2655=AXIS2_PLACEMENT_3D ( 'NONE', #586, #11852, #13669 ) ;
#2660=ORIENTED_EDGE ( 'NONE', *, *, #13454, .F. ) ;
#2668=AXIS2_PLACEMENT_3D ( 'NONE', #19213, #21283, #10439 ) ;
#2681=DIRECTION ( 'NONE',  ( 0.7071067811865416886, 0.000000000000000000, -0.7071067811865532349 ) ) ;
#2687=ADVANCED_FACE ( 'NONE', ( #15260 ), #22593, .F. ) ;
#2690=EDGE_CURVE ( 'NONE', #14056, #3521, #4725, .T. ) ;
#2699=CIRCLE ( 'NONE', #20036, 2.499999999999946709 ) ;
#2708=DIRECTION ( 'NONE',  ( 0.000000000000000000, 0.000000000000000000, -1.000000000000000000 ) ) ;
#2713=ORIENTED_EDGE ( 'NONE', *, *, #21503, .T. ) ;
#2725=EDGE_CURVE ( 'NONE', #15958, #4200, #11618, .T. ) ;
#2732=CARTESIAN_POINT ( 'NONE',  ( -136.9911991620662661, -1072.514904345033301, 29.67072815018525844 ) ) ;
#2738=CARTESIAN_POINT ( 'NONE',  ( 146.4449999999997942, -801.0618695410399823, 30.00000000000641975 ) ) ;
#2740=DIRECTION ( 'NONE',  ( -1.000000000000000000, 1.408839003528726857E-14, 6.982962677686266711E-15 ) ) ;
#2741=CARTESIAN_POINT ( 'NONE',  ( 132.4977819882881249, 80.43276747726562803, 27.56549073392523042 ) ) ;
#2743=DIRECTION ( 'NONE',  ( 0.000000000000000000, 0.000000000000000000, -1.000000000000000000 ) ) ;
#2772=FACE_OUTER_BOUND ( 'NONE', #2800, .T. ) ;
#2800=EDGE_LOOP ( 'NONE', ( #3455, #7439, #7275, #18732 ) ) ;
#2806=EDGE_CURVE ( 'NONE', #590, #13152, #19557, .T. ) ;
#2809=ORIENTED_EDGE ( 'NONE', *, *, #13318, .F. ) ;
#2816=ORIENTED_EDGE ( 'NONE', *, *, #17131, .F. ) ;
#2818=ORIENTED_EDGE ( 'NONE', *, *, #22876, .T. ) ;
#2828=CARTESIAN_POINT ( 'NONE',  ( 146.0000000000002274, -207.9450000000003627, -29.99999999999356604 ) ) ;
#2838=EDGE_CURVE ( 'NONE', #963, #1686, #23641, .T. ) ;
#2840=CARTESIAN_POINT ( 'NONE',  ( 132.2605194320660189, 80.82189108482342021, 27.75096515221180837 ) ) ;
#2841=EDGE_CURVE ( 'NONE', #15576, #12773, #20412, .T. ) ;
#2848=CARTESIAN_POINT ( 'NONE',  ( 155.0000000000000284, -209.9999999999996874, 30.00000000000648015 ) ) ;
#2850=CARTESIAN_POINT ( 'NONE',  ( 121.0905917848625251, -1085.936264790784435, -29.99999999999356604 ) ) ;
#2866=CARTESIAN_POINT ( 'NONE',  ( -134.5482912860058207, -1076.952955187286989, -29.83126738556711288 ) ) ;
#2867=EDGE_LOOP ( 'NONE', ( #2010, #8273 ) ) ;
#2878=DIRECTION ( 'NONE',  ( 1.110223024625155594E-14, 0.000000000000000000, -1.000000000000000000 ) ) ;
#2893=DIRECTION ( 'NONE',  ( 1.000000000000000000, 0.000000000000000000, -0.000000000000000000 ) ) ;
#2896=ORIENTED_EDGE ( 'NONE', *, *, #14175, .F. ) ;
#2902=CONICAL_SURFACE ( 'NONE', #1387, 2.055000000000001492, 0.7853981633974633780 ) ;
#2904=VERTEX_POINT ( 'NONE', #11845 ) ;
#2911=FACE_OUTER_BOUND ( 'NONE', #15555, .T. ) ;
#2913=CARTESIAN_POINT ( 'NONE',  ( 131.8485914335934410, 81.49210221337172300, -31.65735141704659128 ) ) ;
#2933=LINE ( 'NONE', #3298, #4940 ) ;
#2935=DIRECTION ( 'NONE',  ( -1.110223024625157172E-14, 0.000000000000000000, -1.000000000000000000 ) ) ;
#2936=AXIS2_PLACEMENT_3D ( 'NONE', #3907, #20324, #9729 ) ;
#2943=FACE_OUTER_BOUND ( 'NONE', #10466, .T. ) ;
#2946=ORIENTED_EDGE ( 'NONE', *, *, #14978, .T. ) ;
#2951=CARTESIAN_POINT ( 'NONE',  ( -194.7500000000000284, -204.4690652294800657, 30.00000000000675726 ) ) ;
#2952=CARTESIAN_POINT ( 'NONE',  ( 131.6954086522097214, 81.73939080771464205, 31.26048023074364579 ) ) ;
#2955=ORIENTED_EDGE ( 'NONE', *, *, #20821, .F. ) ;
#2964=CARTESIAN_POINT ( 'NONE',  ( 171.6502151485109380, 95.33502053007563859, 32.50000000000675726 ) ) ;
#2974=ORIENTED_EDGE ( 'NONE', *, *, #4137, .T. ) ;
#2978=ORIENTED_EDGE ( 'NONE', *, *, #8640, .T. ) ;
#2988=CIRCLE ( 'NONE', #16132, 2.055000000000001492 ) ;
#2994=CARTESIAN_POINT ( 'NONE',  ( 133.9567665909160326, 77.97815834559297343, -28.74099766568597758 ) ) ;
#3000=CARTESIAN_POINT ( 'NONE',  ( 194.7499999999997442, -801.0618695410399823, 30.00000000000675726 ) ) ;
#3004=CARTESIAN_POINT ( 'NONE',  ( -129.2206655591611764, -1072.408698320350140, -32.05499999999356930 ) ) ;
#3017=CONICAL_SURFACE ( 'NONE', #18819, 2.055000000000001492, 0.7853981633974633780 ) ;
#3018=CARTESIAN_POINT ( 'NONE',  ( -136.3245111336058812, -1073.760768802673056, 27.75040112528352765 ) ) ;
#3029=CARTESIAN_POINT ( 'NONE',  ( 194.7499999999997726, -801.0618695410399823, 27.50000000000675371 ) ) ;
#3041=AXIS2_PLACEMENT_3D ( 'NONE', #19482, #13991, #4770 ) ;
#3051=ORIENTED_EDGE ( 'NONE', *, *, #20882, .F. ) ;
#3069=AXIS2_PLACEMENT_3D ( 'NONE', #19767, #10383, #15579 ) ;
#3072=LINE ( 'NONE', #10339, #13022 ) ;
#3077=DIRECTION ( 'NONE',  ( -1.000000000000000000, 1.408839003528726857E-14, 6.982962677686266711E-15 ) ) ;
#3081=CARTESIAN_POINT ( 'NONE',  ( -146.0000000000001137, -204.4690652294807478, 27.94500000000641649 ) ) ;
#3090=CARTESIAN_POINT ( 'NONE',  ( 131.7919310846380654, 81.58367163796999932, 28.47118012353583794 ) ) ;
#3091=FACE_OUTER_BOUND ( 'NONE', #8718, .T. ) ;
#3098=CARTESIAN_POINT ( 'NONE',  ( -175.1609685624536041, -1088.719770019218913, 32.50000000000675726 ) ) ;
#3101=DIRECTION ( 'NONE',  ( -0.9423651898111408132, -0.3345860861306287348, 6.982962677686266711E-15 ) ) ;
#3103=DIRECTION ( 'NONE',  ( -1.000000000000000000, 1.408839003528726857E-14, 6.982962677686266711E-15 ) ) ;
#3107=DIRECTION ( 'NONE',  ( 0.000000000000000000, 0.000000000000000000, -1.000000000000000000 ) ) ;
#3116=EDGE_CURVE ( 'NONE', #7326, #7198, #10611, .T. ) ;
#3117=EDGE_LOOP ( 'NONE', ( #17465, #3540, #13345, #22736 ) ) ;
#3122=EDGE_CURVE ( 'NONE', #6763, #17109, #2315, .T. ) ;
#3123=CARTESIAN_POINT ( 'NONE',  ( -134.5892462183201701, -1076.881310361371789, -29.34624901867148949 ) ) ;
#3129=EDGE_CURVE ( 'NONE', #13899, #4603, #19279, .T. ) ;
#3131=VERTEX_POINT ( 'NONE', #17477 ) ;
#3133=CARTESIAN_POINT ( 'NONE',  ( 134.0925202534287166, 77.74453171555532549, -30.66034227022097625 ) ) ;
#3137=DIRECTION ( 'NONE',  ( 1.000000000000000000, 0.000000000000000000, 0.000000000000000000 ) ) ;
#3147=EDGE_CURVE ( 'NONE', #4706, #6149, #16156, .T. ) ;
#3149=ORIENTED_EDGE ( 'NONE', *, *, #9898, .T. ) ;
#3150=CYLINDRICAL_SURFACE ( 'NONE', #10428, 2.500000000000002220 ) ;
#3153=CARTESIAN_POINT ( 'NONE',  ( 155.0000000000000284, -209.9999999999996874, 32.50000000000648015 ) ) ;
#3161=DIRECTION ( 'NONE',  ( -0.7232617928448825673, 0.6905739489807055653, 6.982962677686266711E-15 ) ) ;
#3164=CARTESIAN_POINT ( 'NONE',  ( 194.7500000000001990, -210.0000000000003411, -29.99999999999322498 ) ) ;
#3168=PLANE ( 'NONE',  #4606 ) ;
#3174=CARTESIAN_POINT ( 'NONE',  ( -128.5309343563509969, 86.63037569149948069, -32.24903484778816676 ) ) ;
#3180=DIRECTION ( 'NONE',  ( -0.9423651898111408132, -0.3345860861306287348, 6.982962677686266711E-15 ) ) ;
#3188=CARTESIAN_POINT ( 'NONE',  ( -146.0000000000001421, -206.5240652294807546, 30.00000000000641620 ) ) ;
#3194=ORIENTED_EDGE ( 'NONE', *, *, #6533, .T. ) ;
#3199=DIRECTION ( 'NONE',  ( -0.7232617928448825673, 0.6905739489807055653, 6.982962677686266711E-15 ) ) ;
#3201=DIRECTION ( 'NONE',  ( 1.000000000000000000, -0.000000000000000000, -0.000000000000000000 ) ) ;
#3203=VERTEX_POINT ( 'NONE', #23725 ) ;
#3213=ORIENTED_EDGE ( 'NONE', *, *, #12473, .F. ) ;
#3214=DIRECTION ( 'NONE',  ( 0.6964005597823107463, -0.7176533009294141507, 6.982962677686266711E-15 ) ) ;
#3215=CARTESIAN_POINT ( 'NONE',  ( 145.0000000000000284, -500.0000000000000000, 30.00000000000001421 ) ) ;
#3222=EDGE_LOOP ( 'NONE', ( #3855, #5994 ) ) ;
#3225=CARTESIAN_POINT ( 'NONE',  ( -146.0000000000004832, -494.4690652294800657, -27.94499999999356632 ) ) ;
#3227=CARTESIAN_POINT ( 'NONE',  ( -135.7102838464028878, -1074.884883977197887, -27.49999999999352696 ) ) ;
#3235=CARTESIAN_POINT ( 'NONE',  ( 132.8404720734533555, 79.86494211668886578, -32.49999999999351985 ) ) ;
#3242=DIRECTION ( 'NONE',  ( 0.000000000000000000, 0.000000000000000000, -1.000000000000000000 ) ) ;
#3287=CARTESIAN_POINT ( 'NONE',  ( -128.5330911521627399, -1074.345258785412170, -29.99999999999356604 ) ) ;
#3297=CARTESIAN_POINT ( 'NONE',  ( 133.9966253006739407, 77.90961723643370362, 28.88679084683407794 ) ) ;
#3298=CARTESIAN_POINT ( 'NONE',  ( -129.2206655591611764, -1072.408698320350140, -27.94499999999356632 ) ) ;
#3302=DIRECTION ( 'NONE',  ( 0.000000000000000000, 0.000000000000000000, -1.000000000000000000 ) ) ;
#3316=CARTESIAN_POINT ( 'NONE',  ( -158.1195828810602109, 116.4077317428687763, -32.49999999999322853 ) ) ;
#3317=DIRECTION ( 'NONE',  ( 0.000000000000000000, 0.000000000000000000, -1.000000000000000000 ) ) ;
#3325=( LENGTH_UNIT ( ) NAMED_UNIT ( * ) SI_UNIT ( .MILLI., .METRE. ) );
#3335=EDGE_LOOP ( 'NONE', ( #12519, #19471, #19349, #18142 ) ) ;
#3341=DIRECTION ( 'NONE',  ( -1.110223024625155594E-14, 0.000000000000000000, -1.000000000000000000 ) ) ;
#3344=ORIENTED_EDGE ( 'NONE', *, *, #11070, .T. ) ;
#3367=AXIS2_PLACEMENT_3D ( 'NONE', #11000, #18321, #14464 ) ;
#3377=CONICAL_SURFACE ( 'NONE', #15356, 2.055000000000001492, 0.7853981633974633780 ) ;
#3384=CARTESIAN_POINT ( 'NONE',  ( 125.6576742947584364, -1090.747768901066138, -28.46728581292316562 ) ) ;
#3390=ORIENTED_EDGE ( 'NONE', *, *, #3857, .T. ) ;
#3395=ORIENTED_EDGE ( 'NONE', *, *, #22954, .T. ) ;
#3400=EDGE_CURVE ( 'NONE', #907, #20119, #13897, .T. ) ;
#3402=LINE ( 'NONE', #18155, #676 ) ;
#3408=FACE_OUTER_BOUND ( 'NONE', #7905, .T. ) ;
#3414=CARTESIAN_POINT ( 'NONE',  ( 125.6576742947588485, -1090.747768901065228, 31.53271418707689122 ) ) ;
#3416=ADVANCED_FACE ( 'NONE', ( #19381 ), #6719, .F. ) ;
#3418=CARTESIAN_POINT ( 'NONE',  ( 134.1180124237192501, 77.70044921554838879, 30.32918505548582289 ) ) ;
#3426=CARTESIAN_POINT ( 'NONE',  ( -155.0000000000000284, -494.4690652294806341, 30.00000000000648015 ) ) ;
#3433=DIRECTION ( 'NONE',  ( 0.000000000000000000, -1.000000000000000000, 0.000000000000000000 ) ) ;
#3435=CARTESIAN_POINT ( 'NONE',  ( 155.0000000000000284, -500.0000000000000000, -29.99999999999997158 ) ) ;
#3440=CIRCLE ( 'NONE', #20030, 2.499999999999998668 ) ;
#3447=CARTESIAN_POINT ( 'NONE',  ( 146.0000000000002274, -210.0000000000003411, -29.99999999999356604 ) ) ;
#3448=ORIENTED_EDGE ( 'NONE', *, *, #14467, .T. ) ;
#3453=EDGE_CURVE ( 'NONE', #21308, #9451, #23500, .T. ) ;
#3455=ORIENTED_EDGE ( 'NONE', *, *, #23144, .F. ) ;
#3465=CIRCLE ( 'NONE', #5380, 2.499999999999998668 ) ;
#3466=CYLINDRICAL_SURFACE ( 'NONE', #1440, 2.500000000000002220 ) ;
#3481=CARTESIAN_POINT ( 'NONE',  ( -136.1785371930672000, -1074.029921987505077, 32.37408494914631518 ) ) ;
#3486=ORIENTED_EDGE ( 'NONE', *, *, #2725, .T. ) ;
#3496=DIRECTION ( 'NONE',  ( -1.350636282998972974E-14, 0.000000000000000000, -1.000000000000000000 ) ) ;
#3498=EDGE_LOOP ( 'NONE', ( #22994, #15294, #1580, #15933 ) ) ;
#3499=DIRECTION ( 'NONE',  ( -6.753181414994864868E-15, 6.753181414994864868E-15, -1.000000000000000000 ) ) ;
#3500=ORIENTED_EDGE ( 'NONE', *, *, #19418, .T. ) ;
#3502=ORIENTED_EDGE ( 'NONE', *, *, #15244, .T. ) ;
#3503=ADVANCED_FACE ( 'NONE', ( #3091 ), #9228, .F. ) ;
#3510=LINE ( 'NONE', #9435, #20511 ) ;
#3513=DIRECTION ( 'NONE',  ( 0.7071067811865320296, 8.659560562355062281E-17, 0.7071067811865631159 ) ) ;
#3520=CARTESIAN_POINT ( 'NONE',  ( -129.2206655591611764, -1072.408698320350140, -29.99999999999356604 ) ) ;
#3521=VERTEX_POINT ( 'NONE', #12803 ) ;
#3531=CARTESIAN_POINT ( 'NONE',  ( -128.2695163047658298, 87.01699568756195902, 32.42126403526987843 ) ) ;
#3539=EDGE_CURVE ( 'NONE', #15114, #5008, #4223, .T. ) ;
#3540=ORIENTED_EDGE ( 'NONE', *, *, #19795, .T. ) ;
#3547=LINE ( 'NONE', #18279, #18346 ) ;
#3550=LINE ( 'NONE', #3316, #12703 ) ;
#3557=ORIENTED_EDGE ( 'NONE', *, *, #19053, .T. ) ;
#3559=CARTESIAN_POINT ( 'NONE',  ( 124.2735041650576449, -1092.634345841123832, -32.48402282453940160 ) ) ;
#3567=DIRECTION ( 'NONE',  ( 1.000000000000000000, -0.000000000000000000, 6.982962677686266711E-15 ) ) ;
#3571=DIRECTION ( 'NONE',  ( -1.110223024625155594E-14, 0.000000000000000000, -1.000000000000000000 ) ) ;
#3572=EDGE_CURVE ( 'NONE', #15996, #6254, #22032, .T. ) ;
#3579=CARTESIAN_POINT ( 'NONE',  ( 153.5653415408401941, -1122.352966361446079, -29.99999999999322498 ) ) ;
#3588=ORIENTED_EDGE ( 'NONE', *, *, #21314, .T. ) ;
#3604=PRODUCT ( 'belt', 'belt', '', ( #3834 ) ) ;
#3614=CYLINDRICAL_SURFACE ( 'NONE', #20322, 2.500000000000002220 ) ;
#3623=DIRECTION ( 'NONE',  ( -0.7232617928448825673, 0.6905739489807055653, 6.982962677686266711E-15 ) ) ;
#3624=ORIENTED_EDGE ( 'NONE', *, *, #149, .T. ) ;
#3638=ORIENTED_EDGE ( 'NONE', *, *, #20535, .T. ) ;
#3642=CARTESIAN_POINT ( 'NONE',  ( 133.8100684787063983, 78.22965734068104382, 28.34183984639741283 ) ) ;
#3648=ORIENTED_EDGE ( 'NONE', *, *, #9452, .T. ) ;
#3661=CARTESIAN_POINT ( 'NONE',  ( -122.8605704798723082, 82.74225173005861222, 30.00000000000641620 ) ) ;
#3674=DIRECTION ( 'NONE',  ( 0.000000000000000000, -1.000000000000000000, 0.000000000000000000 ) ) ;
#3675=DIRECTION ( 'NONE',  ( 1.110223024625155594E-14, 0.000000000000000000, -1.000000000000000000 ) ) ;
#3682=EDGE_LOOP ( 'NONE', ( #8085, #15317, #11499, #3557 ) ) ;
#3689=CIRCLE ( 'NONE', #11858, 2.055000000000001492 ) ;
#3700=CARTESIAN_POINT ( 'NONE',  ( -136.8329206786529539, -1072.813188689869321, 28.74044610054857074 ) ) ;
#3707=CARTESIAN_POINT ( 'NONE',  ( -127.1852154257917249, 88.59424271557217878, -32.17346063704740544 ) ) ;
#3708=EDGE_CURVE ( 'NONE', #15482, #13840, #19117, .T. ) ;
#3710=EDGE_CURVE ( 'NONE', #17062, #1715, #10615, .T. ) ;
#3717=VECTOR ( 'NONE', #15604, 1000.000000000000114 ) ;
#3722=VECTOR ( 'NONE', #16400, 1000.000000000000000 ) ;
#3728=ORIENTED_EDGE ( 'NONE', *, *, #6097, .T. ) ;
#3747=CARTESIAN_POINT ( 'NONE',  ( -136.5243927815879204, -1073.390114808523549, -28.00764941310471556 ) ) ;
#3756=DIRECTION ( 'NONE',  ( -6.982962677686266711E-15, 0.000000000000000000, 1.000000000000000000 ) ) ;
#3757=DIRECTION ( 'NONE',  ( -1.110223024625157172E-14, 0.000000000000000000, -1.000000000000000000 ) ) ;
#3764=CARTESIAN_POINT ( 'NONE',  ( 145.0000000000000284, -500.0000000000000000, -32.49999999999997158 ) ) ;
#3769=DIRECTION ( 'NONE',  ( 1.000000000000000000, 0.000000000000000000, 0.000000000000000000 ) ) ;
#3772=AXIS2_PLACEMENT_3D ( 'NONE', #1692, #14522, #5096 ) ;
#3785=CARTESIAN_POINT ( 'NONE',  ( 146.0000000000002558, -801.0618695410406644, -32.05499999999356930 ) ) ;
#3792=AXIS2_PLACEMENT_3D ( 'NONE', #15641, #10462, #656 ) ;
#3816=AXIS2_PLACEMENT_3D ( 'NONE', #23080, #1231, #12399 ) ;
#3826=DIRECTION ( 'NONE',  ( 0.000000000000000000, 0.000000000000000000, -1.000000000000000000 ) ) ;
#3834=PRODUCT_CONTEXT ( 'NONE', #9845, 'mechanical' ) ;
#3852=EDGE_CURVE ( 'NONE', #18827, #22831, #11991, .T. ) ;
#3855=ORIENTED_EDGE ( 'NONE', *, *, #19775, .T. ) ;
#3857=EDGE_CURVE ( 'NONE', #11790, #19892, #5369, .T. ) ;
#3869=DIRECTION ( 'NONE',  ( 1.110223024625157172E-14, 0.000000000000000000, -1.000000000000000000 ) ) ;
#3876=EDGE_LOOP ( 'NONE', ( #2660, #20408 ) ) ;
#3879=CARTESIAN_POINT ( 'NONE',  ( -136.3944205523264088, -1073.631384736298514, -27.82770220384456294 ) ) ;
#3882=CARTESIAN_POINT ( 'NONE',  ( -134.6768122279365798, -1076.727833257003567, 28.88700448195638515 ) ) ;
#3886=ADVANCED_FACE ( 'NONE', ( #12877 ), #13139, .F. ) ;
#3898=DIRECTION ( 'NONE',  ( 0.000000000000000000, 0.000000000000000000, -1.000000000000000000 ) ) ;
#3907=CARTESIAN_POINT ( 'NONE',  ( 126.3653543294818178, 77.28387428943173632, -29.99999999999356604 ) ) ;
#3915=ORIENTED_EDGE ( 'NONE', *, *, #15028, .T. ) ;
#3919=CYLINDRICAL_SURFACE ( 'NONE', #19024, 2.500000000000002220 ) ;
#3920=LINE ( 'NONE', #12916, #23067 ) ;
#3925=DIRECTION ( 'NONE',  ( 1.000000000000000000, -0.000000000000000000, 6.982962677686266711E-15 ) ) ;
#3931=B_SPLINE_CURVE_WITH_KNOTS ( 'NONE', 3,
 ( #17164, #9563, #12984, #2307, #13462, #15249, #20775, #2054, #13106, #11653, #144, #3983, #20418, #624, #14769, #18958, #5931, #22102, #507, #7757, #9698, #17052, #5573, #14888, #3747, #3879, #2422, #11163, #18492, #16803, #1949, #22583 ),
 .UNSPECIFIED., .F., .F.,
 ( 4, 2, 2, 2, 2, 2, 2, 2, 2, 2, 2, 2, 2, 2, 2, 4 ),
 ( 0.000000000000000000, 0.0004914281572963174896, 0.0009828563145926349793, 0.001474284471888952361, 0.001965712629185269959, 0.002457140786481587773, 0.002948568943777904721, 0.003931425258370744615, 0.004422853415667163043, 0.004914281572963582340, 0.005405709730260000768, 0.005897137887556419197, 0.006388566044852838494, 0.006879994202149256922, 0.007371422359445676219, 0.007862850516742094648 ),
 .UNSPECIFIED. ) ;
#3945=CARTESIAN_POINT ( 'NONE',  ( 194.7500000000001990, -210.0000000000003411, -29.99999999999322498 ) ) ;
#3951=CARTESIAN_POINT ( 'NONE',  ( -129.2206655591611764, -1072.408698320350140, -29.99999999999356604 ) ) ;
#3966=CARTESIAN_POINT ( 'NONE',  ( -129.3084827928272205, 85.46529914716386145, -29.66799569545555215 ) ) ;
#3969=DIRECTION ( 'NONE',  ( -1.000000000000000000, 1.408839003528726857E-14, 6.982962677686266711E-15 ) ) ;
#3982=VERTEX_POINT ( 'NONE', #5470 ) ;
#3983=CARTESIAN_POINT ( 'NONE',  ( -136.8329206786532097, -1072.813188689868639, -31.25955389945148966 ) ) ;
#3984=CARTESIAN_POINT ( 'NONE',  ( 146.0000000000002274, -210.0000000000003411, -29.99999999999356604 ) ) ;
#3993=CARTESIAN_POINT ( 'NONE',  ( 145.9999999999998010, -801.0618695410399823, 30.00000000000641620 ) ) ;
#3997=DIRECTION ( 'NONE',  ( 0.6964005597823107463, -0.7176533009294141507, 6.982962677686266711E-15 ) ) ;
#3999=CARTESIAN_POINT ( 'NONE',  ( -128.7674363984959598, 86.27842408395231644, 28.00959664470845567 ) ) ;
#4002=CIRCLE ( 'NONE', #1698, 155.0000000000000284 ) ;
#4008=ADVANCED_FACE ( 'NONE', ( #3408 ), #2432, .F. ) ;
#4009=SURFACE_STYLE_USAGE ( .BOTH. , #4270 ) ;
#4014=CARTESIAN_POINT ( 'NONE',  ( 146.4450000000002206, -210.0000000000003411, -29.99999999999356248 ) ) ;
#4018=CIRCLE ( 'NONE', #12573, 2.499999999999998668 ) ;
#4020=CARTESIAN_POINT ( 'NONE',  ( 122.9957307409594449, -1094.324181863848480, 30.65186413114633268 ) ) ;
#4022=ORIENTED_EDGE ( 'NONE', *, *, #6374, .F. ) ;
#4034=DIRECTION ( 'NONE',  ( 1.110223024625155594E-14, 0.000000000000000000, -1.000000000000000000 ) ) ;
#4036=DIRECTION ( 'NONE',  ( 0.6964005597823107463, -0.7176533009294141507, 6.982962677686266711E-15 ) ) ;
#4038=DIRECTION ( 'NONE',  ( -0.000000000000000000, -0.000000000000000000, -1.000000000000000000 ) ) ;
#4042=EDGE_LOOP ( 'NONE', ( #10881, #6091, #18981, #7100 ) ) ;
#4043=DIRECTION ( 'NONE',  ( 1.110223024625155594E-14, 0.000000000000000000, -1.000000000000000000 ) ) ;
#4047=VERTEX_POINT ( 'NONE', #750 ) ;
#4055=DIRECTION ( 'NONE',  ( 1.000000000000000000, 0.000000000000000000, 0.000000000000000000 ) ) ;
#4073=DIRECTION ( 'NONE',  ( -0.5114233182937522049, 0.4883095222350258280, -0.7071067811865532349 ) ) ;
#4079=B_SPLINE_CURVE_WITH_KNOTS ( 'NONE', 3,
 ( #3235, #21619, #10531, #17617, #1205, #14037, #4708, #951, #17864, #6873, #19672, #12234, #19539, #3133, #1071, #8457, #23287, #19416, #12594, #10402, #2994, #12486, #21484, #19787, #8694, #10648, #8576, #6514, #5074, #12118, #21257, #17501 ),
 .UNSPECIFIED., .F., .F.,
 ( 4, 2, 2, 2, 2, 2, 2, 2, 2, 2, 2, 2, 2, 2, 2, 4 ),
 ( 0.000000000000000000, 0.0004914281572963870954, 0.0009828563145927741908, 0.001474284471889161178, 0.001965712629185548382, 0.002457140786481935586, 0.002948568943778322356, 0.003931425258371092427, 0.004422853415667472692, 0.004914281572963852956, 0.005405709730260233221, 0.005897137887556612619, 0.006388566044852993751, 0.006879994202149373149, 0.007371422359445754281, 0.007862850516742132811 ),
 .UNSPECIFIED. ) ;
#4096=EDGE_CURVE ( 'NONE', #17932, #471, #22546, .T. ) ;
#4102=AXIS2_PLACEMENT_3D ( 'NONE', #5130, #7611, #15005 ) ;
#4110=DIRECTION ( 'NONE',  ( -1.350636282998972974E-14, 0.000000000000000000, -1.000000000000000000 ) ) ;
#4113=DIRECTION ( 'NONE',  ( 1.000000000000000000, -0.000000000000000000, 6.982962677686266711E-15 ) ) ;
#4121=ORIENTED_EDGE ( 'NONE', *, *, #15583, .T. ) ;
#4130=VERTEX_POINT ( 'NONE', #21502 ) ;
#4137=EDGE_CURVE ( 'NONE', #12774, #8155, #12192, .T. ) ;
#4146=EDGE_CURVE ( 'NONE', #18827, #22176, #4845, .T. ) ;
#4153=EDGE_LOOP ( 'NONE', ( #2818, #16752 ) ) ;
#4156=EDGE_LOOP ( 'NONE', ( #7443, #19707, #21524, #5570 ) ) ;
#4157=DIRECTION ( 'NONE',  ( 1.000000000000000000, -0.000000000000000000, 6.982962677686266711E-15 ) ) ;
#4180=ORIENTED_EDGE ( 'NONE', *, *, #22954, .F. ) ;
#4189=ORIENTED_EDGE ( 'NONE', *, *, #20979, .F. ) ;
#4200=VERTEX_POINT ( 'NONE', #17636 ) ;
#4214=VERTEX_POINT ( 'NONE', #22946 ) ;
#4217=FACE_OUTER_BOUND ( 'NONE', #8744, .T. ) ;
#4223=CIRCLE ( 'NONE', #10430, 2.055000000000001492 ) ;
#4234=CARTESIAN_POINT ( 'NONE',  ( -146.4450000000000500, -204.4690652294806625, 32.50000000000641620 ) ) ;
#4238=( GEOMETRIC_REPRESENTATION_CONTEXT ( 3 ) GLOBAL_UNCERTAINTY_ASSIGNED_CONTEXT ( ( #15507 ) ) GLOBAL_UNIT_ASSIGNED_CONTEXT ( ( #3325, #21804, #14463 ) ) REPRESENTATION_CONTEXT ( 'NONE', 'WORKASPACE' ) );
#4252=EDGE_CURVE ( 'NONE', #471, #17932, #18306, .T. ) ;
#4266=FACE_BOUND ( 'NONE', #11482, .T. ) ;
#4270=SURFACE_SIDE_STYLE ('',( #9955 ) ) ;
#4282=CARTESIAN_POINT ( 'NONE',  ( 124.0796955067757494, -1092.893784429268635, 32.42079297023032325 ) ) ;
#4313=EDGE_LOOP ( 'NONE', ( #23203, #9087, #2978, #2329 ) ) ;
#4320=UNCERTAINTY_MEASURE_WITH_UNIT (LENGTH_MEASURE( 1.000000000000000082E-05 ), #2444, 'distance_accuracy_value', 'NONE');
#4326=CARTESIAN_POINT ( 'NONE',  ( -145.0000000000000284, 0.000000000000000000, 90.00000000000000000 ) ) ;
#4343=DIRECTION ( 'NONE',  ( 1.000000000000000000, -0.000000000000000000, -0.000000000000000000 ) ) ;
#4359=CARTESIAN_POINT ( 'NONE',  ( 146.4450000000002774, -801.0618695410406644, -32.49999999999356248 ) ) ;
#4364=DIRECTION ( 'NONE',  ( -0.000000000000000000, -0.000000000000000000, -1.000000000000000000 ) ) ;
#4367=VECTOR ( 'NONE', #19599, 1000.000000000000114 ) ;
#4385=CARTESIAN_POINT ( 'NONE',  ( -146.0000000000001421, -786.5240652294805841, 30.00000000000641620 ) ) ;
#4408=CARTESIAN_POINT ( 'NONE',  ( 124.5680376182006768, -1092.237904323006887, -27.49999999999351274 ) ) ;
#4409=CARTESIAN_POINT ( 'NONE',  ( 155.0000000000000284, -210.0000000000003411, -32.49999999999350564 ) ) ;
#4422=VECTOR ( 'NONE', #13159, 999.9999999999998863 ) ;
#4430=CARTESIAN_POINT ( 'NONE',  ( 132.5032837044617793, 80.42329363488335048, 32.42126403526988554 ) ) ;
#4431=CARTESIAN_POINT ( 'NONE',  ( -122.8605704798721945, 82.74225173005939382, -29.99999999999356604 ) ) ;
#4434=ORIENTED_EDGE ( 'NONE', *, *, #12764, .T. ) ;
#4437=EDGE_CURVE ( 'NONE', #12356, #10574, #23342, .T. ) ;
#4444=CARTESIAN_POINT ( 'NONE',  ( -146.0000000000004832, -204.4690652294800657, -27.94499999999356632 ) ) ;
#4450=DIRECTION ( 'NONE',  ( 0.000000000000000000, 0.000000000000000000, -1.000000000000000000 ) ) ;
#4455=ADVANCED_FACE ( 'NONE', ( #4217 ), #18942, .F. ) ;
#4457=CARTESIAN_POINT ( 'NONE',  ( -194.7500000000005116, -494.4690652294794404, -32.49999999999322853 ) ) ;
#4462=CIRCLE ( 'NONE', #17187, 2.499999999999998668 ) ;
#4480=EDGE_LOOP ( 'NONE', ( #1520, #13055, #2946, #5666 ) ) ;
#4487=CARTESIAN_POINT ( 'NONE',  ( -146.4450000000005048, -204.4690652294800088, -27.49999999999356604 ) ) ;
#4500=EDGE_LOOP ( 'NONE', ( #14116, #13758, #6776, #2974 ) ) ;
#4507=DIRECTION ( 'NONE',  ( 6.982962677686266711E-15, -9.837870180509810443E-29, 1.000000000000000000 ) ) ;
#4528=CARTESIAN_POINT ( 'NONE',  ( -146.0000000000004832, -204.4690652294800657, -27.94499999999356632 ) ) ;
#4543=DIRECTION ( 'NONE',  ( -0.7232617928448825673, 0.6905739489807055653, 6.982962677686266711E-15 ) ) ;
#4544=CARTESIAN_POINT ( 'NONE',  ( 131.6528213848851294, 81.80793830425585611, 28.88700448195641357 ) ) ;
#4551=CIRCLE ( 'NONE', #11149, 2.055000000000001492 ) ;
#4556=ORIENTED_EDGE ( 'NONE', *, *, #288, .F. ) ;
#4557=CYLINDRICAL_SURFACE ( 'NONE', #2306, 2.500000000000002220 ) ;
#4560=FACE_OUTER_BOUND ( 'NONE', #13739, .T. ) ;
#4564=ORIENTED_EDGE ( 'NONE', *, *, #5166, .T. ) ;
#4582=ORIENTED_EDGE ( 'NONE', *, *, #12252, .F. ) ;
#4583=ORIENTED_EDGE ( 'NONE', *, *, #3539, .F. ) ;
#4588=VECTOR ( 'NONE', #14718, 1000.000000000000000 ) ;
#4592=AXIS2_PLACEMENT_3D ( 'NONE', #23691, #18371, #10935 ) ;
#4603=VERTEX_POINT ( 'NONE', #22920 ) ;
#4606=AXIS2_PLACEMENT_3D ( 'NONE', #1248, #7269, #21877 ) ;
#4608=EDGE_LOOP ( 'NONE', ( #20905, #572, #9873, #15232 ) ) ;
#4616=DIRECTION ( 'NONE',  ( 6.753181414994864868E-15, 0.000000000000000000, -1.000000000000000000 ) ) ;
#4618=DIRECTION ( 'NONE',  ( 0.9289202219288174023, 0.3702799228849934510, 6.982962677686266711E-15 ) ) ;
#4624=VECTOR ( 'NONE', #19907, 1000.000000000000114 ) ;
#4648=AXIS2_PLACEMENT_3D ( 'NONE', #19889, #23398, #3341 ) ;
#4674=FACE_OUTER_BOUND ( 'NONE', #16028, .T. ) ;
#4681=CARTESIAN_POINT ( 'NONE',  ( -146.0000000000000853, -494.4690652294807478, 30.00000000000641620 ) ) ;
#4684=SHAPE_REPRESENTATION ( 'belt', ( #11210 ), #5408 ) ;
#4689=CARTESIAN_POINT ( 'NONE',  ( -155.0000000000000284, -784.4690652294804067, 30.00000000000648015 ) ) ;
#4690=ORIENTED_EDGE ( 'NONE', *, *, #7220, .F. ) ;
#4701=CARTESIAN_POINT ( 'NONE',  ( -135.3962747006864618, -1075.451122483741301, -27.62619522811935013 ) ) ;
#4706=VERTEX_POINT ( 'NONE', #14817 ) ;
#4708=CARTESIAN_POINT ( 'NONE',  ( 133.4862419878495814, 78.78097527456746718, -32.17346063704739834 ) ) ;
#4719=ORIENTED_EDGE ( 'NONE', *, *, #3453, .T. ) ;
#4723=EDGE_CURVE ( 'NONE', #19341, #22268, #10649, .T. ) ;
#4725=LINE ( 'NONE', #10076, #7330 ) ;
#4726=CARTESIAN_POINT ( 'NONE',  ( -194.7500000000000000, -784.4690652294799520, 32.50000000000675726 ) ) ;
#4729=DIRECTION ( 'NONE',  ( 1.110223024625155594E-14, 0.000000000000000000, -1.000000000000000000 ) ) ;
#4741=FACE_OUTER_BOUND ( 'NONE', #4821, .T. ) ;
#4742=CARTESIAN_POINT ( 'NONE',  ( 126.7787238282395208, 77.44864885511604768, 27.50000000000641975 ) ) ;
#4748=CONICAL_SURFACE ( 'NONE', #18238, 2.055000000000001492, 0.7853981633974633780 ) ;
#4758=DIRECTION ( 'NONE',  ( 6.753181414994864868E-15, 0.000000000000000000, -1.000000000000000000 ) ) ;
#4770=DIRECTION ( 'NONE',  ( -1.350636282998972974E-14, 0.000000000000000000, -1.000000000000000000 ) ) ;
#4771=FACE_BOUND ( 'NONE', #1562, .T. ) ;
#4772=ORIENTED_EDGE ( 'NONE', *, *, #10521, .T. ) ;
#4778=LINE ( 'NONE', #3081, #18840 ) ;
#4783=AXIS2_PLACEMENT_3D ( 'NONE', #23387, #3103, #14247 ) ;
#4784=CARTESIAN_POINT ( 'NONE',  ( 131.5858269427383505, 81.91565353609590261, 30.81384172145501665 ) ) ;
#4796=CYLINDRICAL_SURFACE ( 'NONE', #11636, 2.500000000000002220 ) ;
#4800=DIRECTION ( 'NONE',  ( 1.000000000000000000, 0.000000000000000000, -0.000000000000000000 ) ) ;
#4809=FACE_OUTER_BOUND ( 'NONE', #7971, .T. ) ;
#4812=CARTESIAN_POINT ( 'NONE',  ( -126.8186628169060981, 89.11812652456482908, 28.34183984639740572 ) ) ;
#4814=CARTESIAN_POINT ( 'NONE',  ( -134.5479913728703991, -1076.953479568426019, -30.32849798811268727 ) ) ;
#4821=EDGE_LOOP ( 'NONE', ( #9709, #11517 ) ) ;
#4823=AXIS2_PLACEMENT_3D ( 'NONE', #20542, #15728, #4616 ) ;
#4826=VECTOR ( 'NONE', #13766, 1000.000000000000000 ) ;
#4830=CARTESIAN_POINT ( 'NONE',  ( -155.0000000000000284, -494.4690652294806341, 30.00000000000648015 ) ) ;
#4845=LINE ( 'NONE', #4726, #22143 ) ;
#4862=ORIENTED_EDGE ( 'NONE', *, *, #20361, .F. ) ;
#4867=CARTESIAN_POINT ( 'NONE',  ( 132.8404720734533555, 79.86494211668886578, -32.49999999999351985 ) ) ;
#4877=ORIENTED_EDGE ( 'NONE', *, *, #17263, .T. ) ;
#4887=CARTESIAN_POINT ( 'NONE',  ( -129.2206655591611764, -1072.408698320350140, -29.99999999999356604 ) ) ;
#4905=CARTESIAN_POINT ( 'NONE',  ( -123.1824219776882785, 83.04955713735502343, 30.00000000000641975 ) ) ;
#4917=CARTESIAN_POINT ( 'NONE',  ( -175.1609685624536326, -1088.719770019218913, 30.00000000000675726 ) ) ;
#4919=DIRECTION ( 'NONE',  ( 1.000000000000000000, -0.000000000000000000, 6.982962677686266711E-15 ) ) ;
#4921=AXIS2_PLACEMENT_3D ( 'NONE', #16053, #7204, #6860 ) ;
#4928=ORIENTED_EDGE ( 'NONE', *, *, #3453, .F. ) ;
#4934=VERTEX_POINT ( 'NONE', #6933 ) ;
#4938=VECTOR ( 'NONE', #513, 1000.000000000000000 ) ;
#4940=VECTOR ( 'NONE', #10337, 1000.000000000000000 ) ;
#4941=AXIS2_PLACEMENT_3D ( 'NONE', #19828, #3623, #12759 ) ;
#4948=DIRECTION ( 'NONE',  ( -5.551115123125785858E-15, 5.551115123125785858E-15, -1.000000000000000000 ) ) ;
#4951=CARTESIAN_POINT ( 'NONE',  ( 126.7787238282394640, 77.44864885511604768, 32.50000000000641620 ) ) ;
#4964=CARTESIAN_POINT ( 'NONE',  ( -146.0000000000000568, -204.4690652294807478, 32.05500000000641592 ) ) ;
#4965=ORIENTED_EDGE ( 'NONE', *, *, #12548, .T. ) ;
#4973=ORIENTED_EDGE ( 'NONE', *, *, #10568, .T. ) ;
#5004=EDGE_CURVE ( 'NONE', #1268, #22094, #17809, .T. ) ;
#5008=VERTEX_POINT ( 'NONE', #16001 ) ;
#5009=CARTESIAN_POINT ( 'NONE',  ( -128.9672686250721938, 85.97940096925786690, -28.33934113061009441 ) ) ;
#5026=DIRECTION ( 'NONE',  ( -6.982962677686266711E-15, 0.000000000000000000, 1.000000000000000000 ) ) ;
#5039=CARTESIAN_POINT ( 'NONE',  ( -146.0000000000005116, -204.4690652294800657, -29.99999999999356604 ) ) ;
#5048=EDGE_LOOP ( 'NONE', ( #4928, #7759, #12379, #19509 ) ) ;
#5056=CARTESIAN_POINT ( 'NONE',  ( 171.6502151485116485, 95.33502053007514121, -29.99999999999322498 ) ) ;
#5074=CARTESIAN_POINT ( 'NONE',  ( 133.1760469597745669, 79.30426557766901396, -27.57920702976964122 ) ) ;
#5079=ADVANCED_FACE ( 'NONE', ( #6585 ), #2902, .F. ) ;
#5082=CYLINDRICAL_SURFACE ( 'NONE', #14031, 2.500000000000002220 ) ;
#5096=DIRECTION ( 'NONE',  ( 5.050510105632271307E-15, -4.822252111914687128E-15, 1.000000000000000000 ) ) ;
#5110=DIRECTION ( 'NONE',  ( 1.000000000000000000, -0.000000000000000000, 6.982962677686266711E-15 ) ) ;
#5113=ORIENTED_EDGE ( 'NONE', *, *, #22098, .T. ) ;
#5117=ORIENTED_EDGE ( 'NONE', *, *, #11925, .T. ) ;
#5120=CARTESIAN_POINT ( 'NONE',  ( -127.9021285790837510, 87.55595642181941685, -32.49999999999351985 ) ) ;
#5130=CARTESIAN_POINT ( 'NONE',  ( -146.0000000000000853, -204.4690652294807478, 30.00000000000641620 ) ) ;
#5131=ORIENTED_EDGE ( 'NONE', *, *, #1479, .T. ) ;
#5143=FACE_OUTER_BOUND ( 'NONE', #12319, .T. ) ;
#5151=LINE ( 'NONE', #10249, #9559 ) ;
#5166=EDGE_CURVE ( 'NONE', #1715, #17062, #9285, .T. ) ;
#5175=ORIENTED_EDGE ( 'NONE', *, *, #23379, .F. ) ;
#5179=CARTESIAN_POINT ( 'NONE',  ( -155.0000000000000284, -204.4690652294799520, -29.99999999999350564 ) ) ;
#5183=CARTESIAN_POINT ( 'NONE',  ( -123.1824219776881648, 83.04955713735580503, -29.99999999999356248 ) ) ;
#5186=CARTESIAN_POINT ( 'NONE',  ( -126.5033273815582220, 89.56511165728103663, -29.34813586885359626 ) ) ;
#5190=DIRECTION ( 'NONE',  ( -0.7232617928448825673, 0.6905739489807055653, 6.982962677686265922E-15 ) ) ;
#5198=DIRECTION ( 'NONE',  ( 0.000000000000000000, 0.000000000000000000, 1.000000000000000000 ) ) ;
#5206=EDGE_LOOP ( 'NONE', ( #6622, #21358, #10468, #15696 ) ) ;
#5219=AXIS2_PLACEMENT_3D ( 'NONE', #9427, #4343, #13213 ) ;
#5220=EDGE_LOOP ( 'NONE', ( #16379, #14086, #2626, #6872 ) ) ;
#5229=VERTEX_POINT ( 'NONE', #6194 ) ;
#5248=FACE_OUTER_BOUND ( 'NONE', #1372, .T. ) ;
#5256=ADVANCED_BREP_SHAPE_REPRESENTATION ( '', ( #19781, #11210 ), #5408 ) ;
#5260=DIRECTION ( 'NONE',  ( -0.7232617928448825673, 0.6905739489807055653, 6.982962677686266711E-15 ) ) ;
#5261=AXIS2_PLACEMENT_3D ( 'NONE', #17011, #7818, #5777 ) ;
#5283=FACE_OUTER_BOUND ( 'NONE', #4042, .T. ) ;
#5287=LINE ( 'NONE', #3225, #3722 ) ;
#5292=VECTOR ( 'NONE', #19917, 1000.000000000000114 ) ;
#5295=CARTESIAN_POINT ( 'NONE',  ( -136.8705256357205258, -1072.742444906769151, 31.11216498479345205 ) ) ;
#5297=EDGE_CURVE ( 'NONE', #9785, #20023, #6407, .T. ) ;
#5302=CARTESIAN_POINT ( 'NONE',  ( -126.6049454172958377, 89.42142849841020791, -28.88783501520649111 ) ) ;
#5312=CARTESIAN_POINT ( 'NONE',  ( 119.9257125005558606, -1087.686723660049893, 30.00000000000641975 ) ) ;
#5325=AXIS2_PLACEMENT_3D ( 'NONE', #10960, #9126, #21793 ) ;
#5328=CARTESIAN_POINT ( 'NONE',  ( 126.7787238282401461, 77.44864885511553609, -29.99999999999356248 ) ) ;
#5334=CARTESIAN_POINT ( 'NONE',  ( 146.0000000000001990, -210.0000000000003411, -27.94499999999356632 ) ) ;
#5340=CARTESIAN_POINT ( 'NONE',  ( -135.7895026000614678, -1074.740959209980247, 27.50000000000646239 ) ) ;
#5351=AXIS2_PLACEMENT_3D ( 'NONE', #23010, #6478, #19385 ) ;
#5352=ORIENTED_EDGE ( 'NONE', *, *, #23144, .T. ) ;
#5354=CARTESIAN_POINT ( 'NONE',  ( 125.7666110541943709, -1090.596734011949138, 31.26048023074375237 ) ) ;
#5363=EDGE_CURVE ( 'NONE', #885, #15690, #17732, .T. ) ;
#5364=VECTOR ( 'NONE', #1722, 1000.000000000000114 ) ;
#5369=CIRCLE ( 'NONE', #360, 2.499999999999998668 ) ;
#5380=AXIS2_PLACEMENT_3D ( 'NONE', #5183, #14152, #4948 ) ;
#5384=VECTOR ( 'NONE', #900, 1000.000000000000000 ) ;
#5385=AXIS2_PLACEMENT_3D ( 'NONE', #19975, #20318, #3433 ) ;
#5393=ORIENTED_EDGE ( 'NONE', *, *, #16362, .T. ) ;
#5404=AXIS2_PLACEMENT_3D ( 'NONE', #2848, #16034, #17589 ) ;
#5408=( GEOMETRIC_REPRESENTATION_CONTEXT ( 3 ) GLOBAL_UNCERTAINTY_ASSIGNED_CONTEXT ( ( #4320 ) ) GLOBAL_UNIT_ASSIGNED_CONTEXT ( ( #2444, #15390, #13612 ) ) REPRESENTATION_CONTEXT ( 'NONE', 'WORKASPACE' ) );
#5422=CARTESIAN_POINT ( 'NONE',  ( -136.9913212208047923, -1072.514673757700621, 30.16266818053254539 ) ) ;
#5438=ADVANCED_FACE ( 'NONE', ( #21280 ), #3150, .F. ) ;
#5451=CARTESIAN_POINT ( 'NONE',  ( 125.3881179880844741, -1091.120112697373543, -27.99555145635498477 ) ) ;
#5454=ORIENTED_EDGE ( 'NONE', *, *, #8587, .T. ) ;
#5461=DIRECTION ( 'NONE',  ( 0.7071067811865320296, 8.659560562355062281E-17, 0.7071067811865631159 ) ) ;
#5470=CARTESIAN_POINT ( 'NONE',  ( -146.0000000000000568, -204.4690652294807478, 32.05500000000641592 ) ) ;
#5474=CARTESIAN_POINT ( 'NONE',  ( 125.9168667296001729, -1090.387741168242428, 30.65375098132854959 ) ) ;
#5501=CARTESIAN_POINT ( 'NONE',  ( 153.5653415408401941, -1122.352966361446079, -27.49999999999322498 ) ) ;
#5508=AXIS2_PLACEMENT_3D ( 'NONE', #4830, #12121, #1078 ) ;
#5523=DIRECTION ( 'NONE',  ( -1.000000000000000000, 1.408839003528726857E-14, 6.982962677686266711E-15 ) ) ;
#5531=CARTESIAN_POINT ( 'NONE',  ( -136.1788113199116310, -1074.029417785592614, 27.62610291900644555 ) ) ;
#5538=CYLINDRICAL_SURFACE ( 'NONE', #19375, 155.0000000000000284 ) ;
#5539=AXIS2_PLACEMENT_3D ( 'NONE', #10156, #17498, #6752 ) ;
#5543=B_SPLINE_CURVE_WITH_KNOTS ( 'NONE', 3,
 ( #7005, #9172, #16308, #21729, #9305, #22184, #3707, #18222, #14393, #10897, #16529, #23651, #14497, #21956, #12599, #19910, #1671, #5186, #7460, #5302, #21832, #7358, #9054, #22071, #8950, #11125, #16656, #12714, #16418, #14737, #111, #14610 ),
 .UNSPECIFIED., .F., .F.,
 ( 4, 2, 2, 2, 2, 2, 2, 2, 2, 2, 2, 2, 2, 2, 2, 4 ),
 ( 0.000000000000000000, 0.0004914281572963812407, 0.0009828563145927624815, 0.001474284471889143831, 0.001965712629185524963, 0.002457140786481906095, 0.002948568943778287661, 0.003931425258371062936, 0.004422853415667445803, 0.004914281572963828670, 0.005405709730260211537, 0.005897137887556594404, 0.006388566044852978139, 0.006879994202149361006, 0.007371422359445743873, 0.007862850516742125873 ),
 .UNSPECIFIED. ) ;
#5558=AXIS2_PLACEMENT_3D ( 'NONE', #5312, #9312, #18228 ) ;
#5559=CARTESIAN_POINT ( 'NONE',  ( -129.1735827702798929, 85.66907061909597587, -28.88328940716463222 ) ) ;
#5563=CARTESIAN_POINT ( 'NONE',  ( 125.8126197883818520, -1090.532805371500899, -28.88328940716465354 ) ) ;
#5566=DIRECTION ( 'NONE',  ( -0.7232617928448825673, 0.6905739489807055653, 6.982962677686266711E-15 ) ) ;
#5567=FACE_OUTER_BOUND ( 'NONE', #1695, .T. ) ;
#5570=ORIENTED_EDGE ( 'NONE', *, *, #1479, .F. ) ;
#5573=CARTESIAN_POINT ( 'NONE',  ( -136.6968504244152030, -1073.068359172758846, -28.34359615383088737 ) ) ;
#5594=CARTESIAN_POINT ( 'NONE',  ( 133.4124711242726846, 78.90586732742401921, 27.75040112528346015 ) ) ;
#5598=EDGE_LOOP ( 'NONE', ( #2561, #5131 ) ) ;
#5606=DIRECTION ( 'NONE',  ( 1.000000000000000000, -0.000000000000000000, -0.000000000000000000 ) ) ;
#5622=CARTESIAN_POINT ( 'NONE',  ( 123.4696136271386706, -1093.703085459773547, -31.88829724122655662 ) ) ;
#5623=ADVANCED_FACE ( 'NONE', ( #20894 ), #13933, .F. ) ;
#5624=DIRECTION ( 'NONE',  ( -1.350636282998972974E-14, 0.000000000000000000, -1.000000000000000000 ) ) ;
#5643=EDGE_LOOP ( 'NONE', ( #6395, #18496 ) ) ;
#5644=DIRECTION ( 'NONE',  ( 0.000000000000000000, 0.000000000000000000, -1.000000000000000000 ) ) ;
#5649=DIRECTION ( 'NONE',  ( 1.000000000000000000, -0.000000000000000000, -0.000000000000000000 ) ) ;
#5666=ORIENTED_EDGE ( 'NONE', *, *, #8394, .F. ) ;
#5671=CARTESIAN_POINT ( 'NONE',  ( -145.0000000000000284, 0.000000000000000000, -90.00000000000000000 ) ) ;
#5674=DIRECTION ( 'NONE',  ( -1.110223024625155594E-14, 0.000000000000000000, -1.000000000000000000 ) ) ;
#5696=CARTESIAN_POINT ( 'NONE',  ( -134.5479913728701717, -1076.953479568426701, 29.67150201188731984 ) ) ;
#5711=CARTESIAN_POINT ( 'NONE',  ( -146.0000000000004832, -784.4690652294799520, -27.94499999999356632 ) ) ;
#5740=AXIS2_PLACEMENT_3D ( 'NONE', #9744, #4036, #17098 ) ;
#5746=DIRECTION ( 'NONE',  ( 1.110223024625157172E-14, 0.000000000000000000, -1.000000000000000000 ) ) ;
#5749=DIRECTION ( 'NONE',  ( -1.000000000000000000, 1.408839003528726857E-14, 6.982962677686266711E-15 ) ) ;
#5750=DIRECTION ( 'NONE',  ( 1.000000000000000000, -0.000000000000000000, 6.982962677686266711E-15 ) ) ;
#5755=ORIENTED_EDGE ( 'NONE', *, *, #18667, .F. ) ;
#5765=AXIS2_PLACEMENT_3D ( 'NONE', #2850, #19158, #15573 ) ;
#5773=ORIENTED_EDGE ( 'NONE', *, *, #14805, .F. ) ;
#5777=DIRECTION ( 'NONE',  ( 1.110223024625157172E-14, 0.000000000000000000, -1.000000000000000000 ) ) ;
#5783=EDGE_LOOP ( 'NONE', ( #9715, #9854, #19988, #21303 ) ) ;
#5799=DIRECTION ( 'NONE',  ( -1.000000000000000000, 1.408839003528726857E-14, 6.982962677686266711E-15 ) ) ;
#5802=ORIENTED_EDGE ( 'NONE', *, *, #7660, .T. ) ;
#5805=AXIS2_PLACEMENT_3D ( 'NONE', #9994, #11828, #19373 ) ;
#5812=CARTESIAN_POINT ( 'NONE',  ( -128.0869692137157188, 87.28547799715830990, -27.51562286569268068 ) ) ;
#5824=DIRECTION ( 'NONE',  ( -0.7071067811865416886, 9.961996129952529179E-15, -0.7071067811865532349 ) ) ;
#5843=ORIENTED_EDGE ( 'NONE', *, *, #16315, .F. ) ;
#5852=CARTESIAN_POINT ( 'NONE',  ( 123.1514321905984417, -1094.120844545941964, 28.74044610054851745 ) ) ;
#5858=DIRECTION ( 'NONE',  ( -0.9423651898111409242, -0.3345860861306287903, 6.982962677686267499E-15 ) ) ;
#5859=ORIENTED_EDGE ( 'NONE', *, *, #7296, .F. ) ;
#5860=DIRECTION ( 'NONE',  ( 1.000000000000000000, -0.000000000000000000, 6.982962677686266711E-15 ) ) ;
#5868=EDGE_LOOP ( 'NONE', ( #8382, #17611, #19900, #18241 ) ) ;
#5873=EDGE_LOOP ( 'NONE', ( #6690, #5393 ) ) ;
#5879=CARTESIAN_POINT ( 'NONE',  ( -155.0000000000000284, -1000.000000000000000, 90.00000000000000000 ) ) ;
#5882=EDGE_CURVE ( 'NONE', #11264, #6579, #5543, .T. ) ;
#5886=DIRECTION ( 'NONE',  ( 1.000000000000000000, 0.000000000000000000, 0.000000000000000000 ) ) ;
#5887=EDGE_LOOP ( 'NONE', ( #274, #3648, #716, #11634 ) ) ;
#5923=ORIENTED_EDGE ( 'NONE', *, *, #20310, .T. ) ;
#5929=EDGE_LOOP ( 'NONE', ( #3486, #3638 ) ) ;
#5931=CARTESIAN_POINT ( 'NONE',  ( -136.9835704417553757, -1072.529321614196760, -29.67081494451417001 ) ) ;
#5936=CARTESIAN_POINT ( 'NONE',  ( -135.2464651929976753, -1075.719328653694674, 27.75096515221176219 ) ) ;
#5950=AXIS2_PLACEMENT_3D ( 'NONE', #13132, #16713, #3898 ) ;
#5952=EDGE_LOOP ( 'NONE', ( #20876, #11563 ) ) ;
#5954=( NAMED_UNIT ( * ) PLANE_ANGLE_UNIT ( ) SI_UNIT ( $, .RADIAN. ) );
#5968=CARTESIAN_POINT ( 'NONE',  ( 123.1031131805789016, -1094.184009126530555, 28.88679084683406018 ) ) ;
#5971=DIRECTION ( 'NONE',  ( -1.350636282998972974E-14, 0.000000000000000000, -1.000000000000000000 ) ) ;
#5973=VECTOR ( 'NONE', #8060, 1000.000000000000000 ) ;
#5974=FACE_BOUND ( 'NONE', #12898, .T. ) ;
#5991=LINE ( 'NONE', #20712, #10065 ) ;
#5994=ORIENTED_EDGE ( 'NONE', *, *, #10538, .T. ) ;
#5996=FACE_OUTER_BOUND ( 'NONE', #1396, .T. ) ;
#5998=ORIENTED_EDGE ( 'NONE', *, *, #8394, .T. ) ;
#6000=CARTESIAN_POINT ( 'NONE',  ( 155.0000000000000284, -500.0000000000000000, 32.50000000000001421 ) ) ;
#6005=AXIS2_PLACEMENT_3D ( 'NONE', #7369, #7235, #3499 ) ;
#6011=CARTESIAN_POINT ( 'NONE',  ( 155.0000000000000568, -801.0618695410399823, 30.00000000000648015 ) ) ;
#6016=CARTESIAN_POINT ( 'NONE',  ( 155.0000000000000284, -500.0000000000000000, 30.00000000000001421 ) ) ;
#6019=EDGE_CURVE ( 'NONE', #20774, #9451, #10448, .T. ) ;
#6020=EDGE_CURVE ( 'NONE', #13899, #1268, #8078, .T. ) ;
#6038=DIRECTION ( 'NONE',  ( 1.000000000000000000, -0.000000000000000000, -0.000000000000000000 ) ) ;
#6040=ORIENTED_EDGE ( 'NONE', *, *, #16103, .F. ) ;
#6050=CARTESIAN_POINT ( 'NONE',  ( -135.4738523116355964, -1075.311763300250277, 32.42126403526991396 ) ) ;
#6051=ORIENTED_EDGE ( 'NONE', *, *, #3710, .F. ) ;
#6057=CARTESIAN_POINT ( 'NONE',  ( 146.0000000000002274, -799.0068695410406008, -29.99999999999356604 ) ) ;
#6064=VERTEX_POINT ( 'NONE', #22305 ) ;
#6070=ORIENTED_EDGE ( 'NONE', *, *, #12779, .F. ) ;
#6072=FILL_AREA_STYLE_COLOUR ( '', #19651 ) ;
#6085=CONICAL_SURFACE ( 'NONE', #4941, 2.055000000000001492, 0.7853981633974633780 ) ;
#6086=CARTESIAN_POINT ( 'NONE',  ( -194.7500000000000284, -784.4690652294799520, 30.00000000000675726 ) ) ;
#6087=CARTESIAN_POINT ( 'NONE',  ( 123.8014913250401037, -1093.264216588538829, 27.75040112528339975 ) ) ;
#6091=ORIENTED_EDGE ( 'NONE', *, *, #21075, .F. ) ;
#6095=EDGE_CURVE ( 'NONE', #22094, #18595, #10064, .T. ) ;
#6097=EDGE_CURVE ( 'NONE', #22916, #15482, #12799, .T. ) ;
#6101=LINE ( 'NONE', #22631, #16930 ) ;
#6112=ORIENTED_EDGE ( 'NONE', *, *, #3116, .F. ) ;
#6114=DIRECTION ( 'NONE',  ( -0.9423651898111408132, -0.3345860861306287348, 6.982962677686266711E-15 ) ) ;
#6127=CARTESIAN_POINT ( 'NONE',  ( 126.3653543294811499, 77.28387428943223370, 30.00000000000641620 ) ) ;
#6148=AXIS2_PLACEMENT_3D ( 'NONE', #6127, #23139, #2743 ) ;
#6149=VERTEX_POINT ( 'NONE', #2622 ) ;
#6151=CARTESIAN_POINT ( 'NONE',  ( -126.6510233831472050, 89.35617925171740694, 31.25900233431401531 ) ) ;
#6167=ADVANCED_FACE ( 'NONE', ( #4560 ), #4796, .F. ) ;
#6175=EDGE_CURVE ( 'NONE', #22916, #23140, #19512, .T. ) ;
#6178=CYLINDRICAL_SURFACE ( 'NONE', #4648, 2.500000000000002220 ) ;
#6184=ORIENTED_EDGE ( 'NONE', *, *, #2841, .T. ) ;
#6194=CARTESIAN_POINT ( 'NONE',  ( 119.9257125005557043, -1087.686723660050802, -27.49999999999356248 ) ) ;
#6218=CARTESIAN_POINT ( 'NONE',  ( 123.7141469857653391, -1093.380023028671530, 27.82653936295259811 ) ) ;
#6232=ADVANCED_FACE ( 'NONE', ( #19392 ), #11851, .F. ) ;
#6245=DIRECTION ( 'NONE',  ( 0.000000000000000000, 0.000000000000000000, -1.000000000000000000 ) ) ;
#6248=EDGE_CURVE ( 'NONE', #45, #493, #1405, .T. ) ;
#6250=ORIENTED_EDGE ( 'NONE', *, *, #21144, .F. ) ;
#6254=VERTEX_POINT ( 'NONE', #10975 ) ;
#6261=CARTESIAN_POINT ( 'NONE',  ( 126.7787238282394924, 77.44864885511604768, 30.00000000000641975 ) ) ;
#6264=AXIS2_PLACEMENT_3D ( 'NONE', #17505, #23294, #21262 ) ;
#6265=EDGE_LOOP ( 'NONE', ( #8209, #7833 ) ) ;
#6267=CARTESIAN_POINT ( 'NONE',  ( 124.4701338314433485, -1092.369831568443260, -27.49999999999351985 ) ) ;
#6269=EDGE_CURVE ( 'NONE', #6379, #11094, #16152, .T. ) ;
#6272=CARTESIAN_POINT ( 'NONE',  ( 126.3653543294811499, 77.28387428943223370, 32.05500000000640171 ) ) ;
#6274=CARTESIAN_POINT ( 'NONE',  ( -126.8176664439037182, 89.11954614941086561, 31.65640384616917657 ) ) ;
#6306=CARTESIAN_POINT ( 'NONE',  ( 155.0000000000000284, -210.0000000000003411, -27.49999999999350209 ) ) ;
#6311=ORIENTED_EDGE ( 'NONE', *, *, #3400, .F. ) ;
#6318=EDGE_CURVE ( 'NONE', #9451, #20774, #7692, .T. ) ;
#6346=AXIS2_PLACEMENT_3D ( 'NONE', #9368, #20456, #184 ) ;
#6354=LINE ( 'NONE', #11957, #4826 ) ;
#6356=CIRCLE ( 'NONE', #21383, 2.500000000000002220 ) ;
#6366=ORIENTED_EDGE ( 'NONE', *, *, #16200, .T. ) ;
#6374=EDGE_CURVE ( 'NONE', #2426, #11453, #82, .T. ) ;
#6379=VERTEX_POINT ( 'NONE', #2223 ) ;
#6383=AXIS2_PLACEMENT_3D ( 'NONE', #10030, #2628, #22803 ) ;
#6395=ORIENTED_EDGE ( 'NONE', *, *, #18076, .T. ) ;
#6407=CIRCLE ( 'NONE', #16815, 2.499999999999998668 ) ;
#6419=CARTESIAN_POINT ( 'NONE',  ( 119.6158142514525622, -1087.367367941136990, -29.99999999999356604 ) ) ;
#6436=DIRECTION ( 'NONE',  ( -1.000000000000000000, 1.408839003528726857E-14, 6.982962677686266711E-15 ) ) ;
#6458=DIRECTION ( 'NONE',  ( 0.000000000000000000, 0.000000000000000000, -1.000000000000000000 ) ) ;
#6470=FACE_OUTER_BOUND ( 'NONE', #18190, .T. ) ;
#6471=CARTESIAN_POINT ( 'NONE',  ( -146.4450000000001069, -494.4690652294807478, 27.50000000000642331 ) ) ;
#6473=CARTESIAN_POINT ( 'NONE',  ( 131.5246926503482996, 82.01375679560405274, 30.33200430454443719 ) ) ;
#6478=DIRECTION ( 'NONE',  ( 1.000000000000000000, 0.000000000000000000, -0.000000000000000000 ) ) ;
#6485=DIRECTION ( 'NONE',  ( 0.9289202219288174023, 0.3702799228849933955, 6.982962677686265922E-15 ) ) ;
#6497=VECTOR ( 'NONE', #22041, 1000.000000000000114 ) ;
#6500=DIRECTION ( 'NONE',  ( -1.000000000000000000, 1.408839003528726857E-14, 6.982962677686266711E-15 ) ) ;
#6503=CARTESIAN_POINT ( 'NONE',  ( -126.7571989378452599, 89.20549877611294676, 31.53022738271492997 ) ) ;
#6505=CARTESIAN_POINT ( 'NONE',  ( -134.5566256099407099, -1076.938388239962933, -29.66799569545555215 ) ) ;
#6514=CARTESIAN_POINT ( 'NONE',  ( 133.2563391751591837, 79.16925799295223953, -27.62591505085368127 ) ) ;
#6520=CARTESIAN_POINT ( 'NONE',  ( -146.0000000000000853, -204.4690652294807478, 30.00000000000641620 ) ) ;
#6533=EDGE_CURVE ( 'NONE', #14975, #4130, #18469, .T. ) ;
#6541=CIRCLE ( 'NONE', #5385, 2.500000000000002220 ) ;
#6559=AXIS2_PLACEMENT_3D ( 'NONE', #6664, #12393, #23315 ) ;
#6576=DIRECTION ( 'NONE',  ( 1.000000000000000000, 0.000000000000000000, -0.000000000000000000 ) ) ;
#6579=VERTEX_POINT ( 'NONE', #6785 ) ;
#6585=FACE_OUTER_BOUND ( 'NONE', #20085, .T. ) ;
#6592=PLANE ( 'NONE',  #22479 ) ;
#6593=ORIENTED_EDGE ( 'NONE', *, *, #7220, .T. ) ;
#6595=CARTESIAN_POINT ( 'NONE',  ( 145.9999999999998010, -799.0068695410399187, 30.00000000000641620 ) ) ;
#6596=DIRECTION ( 'NONE',  ( 0.9289202219288174023, 0.3702799228849934510, 6.982962677686266711E-15 ) ) ;
#6606=CARTESIAN_POINT ( 'NONE',  ( 132.6714475832642677, 80.14557597091010166, 32.48437713430730156 ) ) ;
#6613=LINE ( 'NONE', #1034, #1685 ) ;
#6615=DIRECTION ( 'NONE',  ( -1.110223024625155594E-14, 0.000000000000000000, -1.000000000000000000 ) ) ;
#6616=DIRECTION ( 'NONE',  ( 0.7071067811865416886, 0.000000000000000000, -0.7071067811865532349 ) ) ;
#6622=ORIENTED_EDGE ( 'NONE', *, *, #21314, .F. ) ;
#6623=VERTEX_POINT ( 'NONE', #3153 ) ;
#6631=CARTESIAN_POINT ( 'NONE',  ( -126.4656051290186980, 89.61836744852057279, 30.32918505548581933 ) ) ;
#6641=ORIENTED_EDGE ( 'NONE', *, *, #18645, .F. ) ;
#6658=EDGE_CURVE ( 'NONE', #18017, #9785, #7025, .T. ) ;
#6664=CARTESIAN_POINT ( 'NONE',  ( -146.4450000000005332, -204.4690652294800657, -29.99999999999356248 ) ) ;
#6670=EDGE_CURVE ( 'NONE', #8689, #22922, #10900, .T. ) ;
#6682=CARTESIAN_POINT ( 'NONE',  ( 194.7500000000001990, -801.0618695410406644, -29.99999999999322498 ) ) ;
#6683=ORIENTED_EDGE ( 'NONE', *, *, #17012, .F. ) ;
#6686=ORIENTED_EDGE ( 'NONE', *, *, #149, .F. ) ;
#6690=ORIENTED_EDGE ( 'NONE', *, *, #17142, .T. ) ;
#6692=EDGE_LOOP ( 'NONE', ( #14133, #15065, #8571, #3395 ) ) ;
#6702=EDGE_CURVE ( 'NONE', #13026, #10799, #3440, .T. ) ;
#6710=EDGE_LOOP ( 'NONE', ( #9697, #8958, #14457, #2955 ) ) ;
#6719=PLANE ( 'NONE',  #23487 ) ;
#6728=CYLINDRICAL_SURFACE ( 'NONE', #6865, 2.500000000000002220 ) ;
#6729=DIRECTION ( 'NONE',  ( 0.000000000000000000, 0.000000000000000000, 1.000000000000000000 ) ) ;
#6741=VECTOR ( 'NONE', #12249, 1000.000000000000000 ) ;
#6748=CARTESIAN_POINT ( 'NONE',  ( -134.9759958199652203, -1076.200356551567211, -31.88744336596582940 ) ) ;
#6752=DIRECTION ( 'NONE',  ( 1.000000000000000000, 0.000000000000000000, 0.000000000000000000 ) ) ;
#6763=VERTEX_POINT ( 'NONE', #20060 ) ;
#6764=CARTESIAN_POINT ( 'NONE',  ( -194.7500000000005116, -204.4690652294793836, -32.49999999999322853 ) ) ;
#6766=EDGE_CURVE ( 'NONE', #21251, #18595, #3510, .T. ) ;
#6773=AXIS2_PLACEMENT_3D ( 'NONE', #21845, #20042, #3496 ) ;
#6776=ORIENTED_EDGE ( 'NONE', *, *, #8577, .T. ) ;
#6778=CARTESIAN_POINT ( 'NONE',  ( -136.1034519145105719, -1074.167893320493249, 32.42079297023033035 ) ) ;
#6785=CARTESIAN_POINT ( 'NONE',  ( -127.9021285790837510, 87.55595642181940264, -27.49999999999351985 ) ) ;
#6805=FACE_OUTER_BOUND ( 'NONE', #5952, .T. ) ;
#6810=CARTESIAN_POINT ( 'NONE',  ( -127.9949300873392275, 87.42039156791001631, -27.49999999999351985 ) ) ;
#6821=FACE_OUTER_BOUND ( 'NONE', #5643, .T. ) ;
#6825=PLANE ( 'NONE',  #15465 ) ;
#6829=ADVANCED_FACE ( 'NONE', ( #17045 ), #22457, .F. ) ;
#6835=DIRECTION ( 'NONE',  ( -1.350636282998972974E-14, 0.000000000000000000, -1.000000000000000000 ) ) ;
#6836=ORIENTED_EDGE ( 'NONE', *, *, #19483, .F. ) ;
#6838=CARTESIAN_POINT ( 'NONE',  ( -146.0000000000000568, -494.4690652294807478, 32.05500000000641592 ) ) ;
#6844=DIRECTION ( 'NONE',  ( 0.000000000000000000, -1.000000000000000000, 0.000000000000000000 ) ) ;
#6857=AXIS2_PLACEMENT_3D ( 'NONE', #6595, #22992, #5026 ) ;
#6860=DIRECTION ( 'NONE',  ( 0.000000000000000000, 0.000000000000000000, -1.000000000000000000 ) ) ;
#6863=CIRCLE ( 'NONE', #9478, 2.055000000000001492 ) ;
#6865=AXIS2_PLACEMENT_3D ( 'NONE', #4917, #3101, #12457 ) ;
#6872=ORIENTED_EDGE ( 'NONE', *, *, #10521, .F. ) ;
#6873=CARTESIAN_POINT ( 'NONE',  ( 133.8100684787067962, 78.22965734068039012, -31.65816015360256586 ) ) ;
#6886=LINE ( 'NONE', #14293, #22619 ) ;
#6902=EDGE_CURVE ( 'NONE', #10962, #11798, #12866, .T. ) ;
#6903=VECTOR ( 'NONE', #12316, 1000.000000000000000 ) ;
#6917=AXIS2_PLACEMENT_3D ( 'NONE', #22153, #5749, #5624 ) ;
#6922=CARTESIAN_POINT ( 'NONE',  ( -155.0000000000000284, -204.4690652294799520, -29.99999999999350564 ) ) ;
#6926=EDGE_CURVE ( 'NONE', #10443, #11094, #2126, .T. ) ;
#6931=ORIENTED_EDGE ( 'NONE', *, *, #20535, .F. ) ;
#6932=CARTESIAN_POINT ( 'NONE',  ( -129.1746529357993722, 85.66745698985798185, -31.11299551804356156 ) ) ;
#6933=CARTESIAN_POINT ( 'NONE',  ( -146.4450000000005048, -784.4690652294799520, -27.49999999999356604 ) ) ;
#6936=EDGE_LOOP ( 'NONE', ( #512, #21864 ) ) ;
#6950=ORIENTED_EDGE ( 'NONE', *, *, #10538, .F. ) ;
#6960=VECTOR ( 'NONE', #6485, 1000.000000000000114 ) ;
#6967=DIRECTION ( 'NONE',  ( 0.9289202219288174023, 0.3702799228849933955, 6.982962677686265922E-15 ) ) ;
#6976=CARTESIAN_POINT ( 'NONE',  ( -135.7895026000614109, -1074.740959209980247, 32.50000000000646594 ) ) ;
#6980=FACE_BOUND ( 'NONE', #14483, .T. ) ;
#6981=CARTESIAN_POINT ( 'NONE',  ( -175.1609685624542863, -1088.719770019218458, -32.49999999999322853 ) ) ;
#7002=DIRECTION ( 'NONE',  ( -1.350636282998972974E-14, 0.000000000000000000, -1.000000000000000000 ) ) ;
#7005=CARTESIAN_POINT ( 'NONE',  ( -127.9021285790837510, 87.55595642181941685, -32.49999999999351985 ) ) ;
#7007=CARTESIAN_POINT ( 'NONE',  ( 0.000000000000000000, 0.000000000000000000, 90.00000000000000000 ) ) ;
#7013=ORIENTED_EDGE ( 'NONE', *, *, #21144, .T. ) ;
#7025=LINE ( 'NONE', #9863, #15814 ) ;
#7028=DIRECTION ( 'NONE',  ( 0.000000000000000000, 0.000000000000000000, -1.000000000000000000 ) ) ;
#7029=AXIS2_PLACEMENT_3D ( 'NONE', #11647, #6038, #18824 ) ;
#7034=DIRECTION ( 'NONE',  ( 0.000000000000000000, 5.551115123125777969E-15, -1.000000000000000000 ) ) ;
#7040=ORIENTED_EDGE ( 'NONE', *, *, #15096, .T. ) ;
#7041=DIRECTION ( 'NONE',  ( 6.580500949201931673E-15, 2.336402151923303105E-15, 1.000000000000000000 ) ) ;
#7050=CARTESIAN_POINT ( 'NONE',  ( -146.0000000000001137, -494.4690652294807478, 27.94500000000641649 ) ) ;
#7059=ADVANCED_FACE ( 'NONE', ( #15674 ), #14391, .F. ) ;
#7067=CARTESIAN_POINT ( 'NONE',  ( 194.7499999999997158, -801.0618695410399823, 32.50000000000675726 ) ) ;
#7069=DIRECTION ( 'NONE',  ( -1.000000000000000000, 1.408839003528726857E-14, 6.982962677686266711E-15 ) ) ;
#7072=DIRECTION ( 'NONE',  ( 0.000000000000000000, 0.000000000000000000, -1.000000000000000000 ) ) ;
#7085=EDGE_LOOP ( 'NONE', ( #11423, #15351, #11328, #22585 ) ) ;
#7092=CARTESIAN_POINT ( 'NONE',  ( 126.3653543294818178, 77.28387428943173632, -27.94499999999356632 ) ) ;
#7093=DIRECTION ( 'NONE',  ( -1.000000000000000000, 1.408839003528726857E-14, 6.982962677686266711E-15 ) ) ;
#7099=CARTESIAN_POINT ( 'NONE',  ( 119.9257125005557043, -1087.686723660050802, -29.99999999999356248 ) ) ;
#7100=ORIENTED_EDGE ( 'NONE', *, *, #7660, .F. ) ;
#7109=ORIENTED_EDGE ( 'NONE', *, *, #12162, .T. ) ;
#7113=AXIS2_PLACEMENT_3D ( 'NONE', #22377, #14911, #7283 ) ;
#7114=FACE_OUTER_BOUND ( 'NONE', #10569, .T. ) ;
#7117=EDGE_LOOP ( 'NONE', ( #13046, #10761 ) ) ;
#7125=AXIS2_PLACEMENT_3D ( 'NONE', #2951, #8539, #12314 ) ;
#7130=ADVANCED_FACE ( 'NONE', ( #10161 ), #8581, .F. ) ;
#7147=AXIS2_PLACEMENT_3D ( 'NONE', #9610, #192, #18633 ) ;
#7185=CARTESIAN_POINT ( 'NONE',  ( 123.3278826340502548, -1093.889547229276104, -31.65816015360254454 ) ) ;
#7198=VERTEX_POINT ( 'NONE', #17620 ) ;
#7204=DIRECTION ( 'NONE',  ( 0.9289202219288174023, 0.3702799228849934510, 6.982962677686266711E-15 ) ) ;
#7208=AXIS2_PLACEMENT_3D ( 'NONE', #12340, #3214, #8432 ) ;
#7220=EDGE_CURVE ( 'NONE', #16055, #6064, #21323, .T. ) ;
#7223=ADVANCED_FACE ( 'NONE', ( #8335 ), #5082, .F. ) ;
#7224=ORIENTED_EDGE ( 'NONE', *, *, #3857, .F. ) ;
#7231=CIRCLE ( 'NONE', #10756, 145.0000000000000284 ) ;
#7235=DIRECTION ( 'NONE',  ( -0.7232617928448825673, 0.6905739489807055653, 6.982962677686266711E-15 ) ) ;
#7241=B_SPLINE_CURVE_WITH_KNOTS ( 'NONE', 3,
 ( #8686, #3227, #12112, #23035, #4701, #19408, #17495, #23404, #10395, #834, #14269, #21610, #3123, #6505, #2866, #4814, #19778, #17745, #8570, #17396, #15939, #6748, #8323, #16056, #944, #8448, #15702, #17609 ),
 .UNSPECIFIED., .F., .F.,
 ( 4, 2, 2, 2, 2, 2, 2, 2, 2, 2, 2, 2, 2, 4 ),
 ( 0.007862850516742094648, 0.008354729399060815617, 0.008846608281379538322, 0.009830366046016980261, 0.01032224492833550521, 0.01081412381065403015, 0.01130600269297255510, 0.01179788157529108178, 0.01278163933992811953, 0.01327351822224664274, 0.01376539710456516769, 0.01425727598688369263, 0.01474915486920221758, 0.01573291263383921890 ),
 .UNSPECIFIED. ) ;
#7247=PLANE ( 'NONE',  #3772 ) ;
#7249=AXIS2_PLACEMENT_3D ( 'NONE', #2738, #13763, #22998 ) ;
#7255=ORIENTED_EDGE ( 'NONE', *, *, #3539, .T. ) ;
#7261=ORIENTED_EDGE ( 'NONE', *, *, #20979, .T. ) ;
#7269=DIRECTION ( 'NONE',  ( -1.000000000000000000, 0.000000000000000000, -6.982962677686266711E-15 ) ) ;
#7275=ORIENTED_EDGE ( 'NONE', *, *, #22002, .F. ) ;
#7276=CARTESIAN_POINT ( 'NONE',  ( 124.8578076529642971, -1091.845273256945802, 32.42126403526987133 ) ) ;
#7282=ADVANCED_FACE ( 'NONE', ( #2772 ), #113, .F. ) ;
#7283=DIRECTION ( 'NONE',  ( 6.753181414994864868E-15, 0.000000000000000000, -1.000000000000000000 ) ) ;
#7296=EDGE_CURVE ( 'NONE', #23044, #4047, #1786, .T. ) ;
#7301=CARTESIAN_POINT ( 'NONE',  ( -122.8605704798721803, 82.74225173005937961, -27.94499999999356632 ) ) ;
#7305=CIRCLE ( 'NONE', #13910, 2.055000000000001492 ) ;
#7312=VECTOR ( 'NONE', #9127, 1000.000000000000114 ) ;
#7313=VECTOR ( 'NONE', #15694, 1000.000000000000000 ) ;
#7315=ORIENTED_EDGE ( 'NONE', *, *, #19836, .F. ) ;
#7319=CARTESIAN_POINT ( 'NONE',  ( 122.9459112154324032, -1094.389103796012705, -29.83733181946741908 ) ) ;
#7326=VERTEX_POINT ( 'NONE', #14856 ) ;
#7330=VECTOR ( 'NONE', #2681, 1000.000000000000114 ) ;
#7331=AXIS2_PLACEMENT_3D ( 'NONE', #10687, #23576, #8974 ) ;
#7336=ADVANCED_FACE ( 'NONE', ( #11127, #16532, #18117, #14499, #23655 ), #5538, .T. ) ;
#7350=VECTOR ( 'NONE', #3513, 1000.000000000000000 ) ;
#7358=CARTESIAN_POINT ( 'NONE',  ( -126.7571989378447910, 89.20549877611344414, -28.46977261728505937 ) ) ;
#7367=DIRECTION ( 'NONE',  ( 1.000000000000000000, -0.000000000000000000, 6.982962677686266711E-15 ) ) ;
#7369=CARTESIAN_POINT ( 'NONE',  ( -122.8605704798721945, 82.74225173005939382, -29.99999999999356604 ) ) ;
#7376=CARTESIAN_POINT ( 'NONE',  ( -129.2722218393572859, 85.52013646629116295, -29.34624901867147528 ) ) ;
#7383=LINE ( 'NONE', #5334, #7350 ) ;
#7403=CARTESIAN_POINT ( 'NONE',  ( 125.5963796795001031, -1090.832610870656481, 28.34264858295336964 ) ) ;
#7407=CARTESIAN_POINT ( 'NONE',  ( -128.9689330775211999, 85.97690438148575254, 28.34264858295340517 ) ) ;
#7419=FACE_OUTER_BOUND ( 'NONE', #16199, .T. ) ;
#7422=DIRECTION ( 'NONE',  ( -1.000000000000000000, 1.408839003528726857E-14, 6.982962677686266711E-15 ) ) ;
#7428=DIRECTION ( 'NONE',  ( 1.000000000000000000, 0.000000000000000000, -0.000000000000000000 ) ) ;
#7439=ORIENTED_EDGE ( 'NONE', *, *, #1857, .T. ) ;
#7443=ORIENTED_EDGE ( 'NONE', *, *, #12162, .F. ) ;
#7460=CARTESIAN_POINT ( 'NONE',  ( -126.5312127422330519, 89.52572971382308253, -29.19154146838982200 ) ) ;
#7470=CARTESIAN_POINT ( 'NONE',  ( -194.7500000000000568, -494.4690652294800657, 27.50000000000675371 ) ) ;
#7480=VECTOR ( 'NONE', #597, 1000.000000000000000 ) ;
#7506=CARTESIAN_POINT ( 'NONE',  ( 119.6158142514527185, -1087.367367941136308, 32.05500000000640881 ) ) ;
#7511=CIRCLE ( 'NONE', #23714, 2.055000000000001492 ) ;
#7525=CARTESIAN_POINT ( 'NONE',  ( 119.6158142514525480, -1087.367367941136990, -27.94499999999356632 ) ) ;
#7527=CARTESIAN_POINT ( 'NONE',  ( 131.5507733270954134, 81.97201125882388340, -30.65604281379822638 ) ) ;
#7532=ADVANCED_FACE ( 'NONE', ( #11853 ), #15103, .F. ) ;
#7546=LINE ( 'NONE', #14934, #4422 ) ;
#7560=CARTESIAN_POINT ( 'NONE',  ( -146.0000000000000853, -204.4690652294807478, 30.00000000000641620 ) ) ;
#7563=CARTESIAN_POINT ( 'NONE',  ( 145.0000000000000284, -500.0000000000000000, 32.50000000000001421 ) ) ;
#7575=CARTESIAN_POINT ( 'NONE',  ( -136.8330323738929621, -1072.812977866783285, 31.25900233431395137 ) ) ;
#7576=CARTESIAN_POINT ( 'NONE',  ( 119.6158142514525764, -1087.367367941136990, -32.05499999999356930 ) ) ;
#7577=ORIENTED_EDGE ( 'NONE', *, *, #3147, .F. ) ;
#7583=CARTESIAN_POINT ( 'NONE',  ( -175.1609685624542578, -1088.719770019218458, -29.99999999999322498 ) ) ;
#7587=DIRECTION ( 'NONE',  ( -1.110223024625157172E-14, 0.000000000000000000, -1.000000000000000000 ) ) ;
#7600=DIRECTION ( 'NONE',  ( -0.9423651898111408132, -0.3345860861306287348, 6.982962677686266711E-15 ) ) ;
#7611=DIRECTION ( 'NONE',  ( -1.000000000000000000, 1.408839003528726857E-14, 6.982962677686266711E-15 ) ) ;
#7621=CARTESIAN_POINT ( 'NONE',  ( -135.0351526491285199, -1076.095746396249979, 32.00444854364506853 ) ) ;
#7633=CARTESIAN_POINT ( 'NONE',  ( 125.2216071840750402, -1091.349008980711915, 32.18904844917292252 ) ) ;
#7635=CARTESIAN_POINT ( 'NONE',  ( -129.0269476471448513, 85.88978664864519885, 31.53271418707683083 ) ) ;
#7646=CARTESIAN_POINT ( 'NONE',  ( 131.6954086522101193, 81.73939080771404520, -28.73951976925631868 ) ) ;
#7653=B_SPLINE_CURVE_WITH_KNOTS ( 'NONE', 3,
 ( #483, #7842, #15224, #20507, #16899, #365, #13573, #17141, #19051, #4812, #21355, #17607, #17493, #23167, #598, #20886, #6631, #10268, #14027, #22681, #6151, #6503, #6274, #8321, #23031, #13682, #11745, #7961, #15343, #19406, #22914, #941 ),
 .UNSPECIFIED., .F., .F.,
 ( 4, 2, 2, 2, 2, 2, 2, 2, 2, 2, 2, 2, 2, 2, 2, 4 ),
 ( 0.000000000000000000, 0.0004914281572963851439, 0.0009828563145927702877, 0.001474284471889155540, 0.001965712629185540575, 0.002457140786481926045, 0.002948568943778311080, 0.003931425258371084620, 0.004422853415667466620, 0.004914281572963847752, 0.005405709730260229752, 0.005897137887556611752, 0.006388566044852992884, 0.006879994202149374016, 0.007371422359445756016, 0.007862850516742138016 ),
 .UNSPECIFIED. ) ;
#7655=FACE_OUTER_BOUND ( 'NONE', #5868, .T. ) ;
#7656=CARTESIAN_POINT ( 'NONE',  ( 123.3268328482426881, -1093.890927824661276, 31.65640384616908420 ) ) ;
#7660=EDGE_CURVE ( 'NONE', #22176, #19928, #23254, .T. ) ;
#7672=AXIS2_PLACEMENT_3D ( 'NONE', #7998, #634, #18968 ) ;
#7673=AXIS2_PLACEMENT_3D ( 'NONE', #17282, #726, #10057 ) ;
#7676=CYLINDRICAL_SURFACE ( 'NONE', #8254, 2.500000000000002220 ) ;
#7684=EDGE_LOOP ( 'NONE', ( #17817, #1233, #2896, #8593 ) ) ;
#7685=ORIENTED_EDGE ( 'NONE', *, *, #20929, .T. ) ;
#7692=CIRCLE ( 'NONE', #11571, 2.499999999999946709 ) ;
#7703=EDGE_CURVE ( 'NONE', #14948, #22288, #20118, .T. ) ;
#7708=CARTESIAN_POINT ( 'NONE',  ( 0.000000000000000000, 0.000000000000000000, -90.00000000000000000 ) ) ;
#7715=VECTOR ( 'NONE', #19064, 1000.000000000000114 ) ;
#7751=CARTESIAN_POINT ( 'NONE',  ( -146.0000000000005116, -494.4690652294800657, -29.99999999999356604 ) ) ;
#7757=CARTESIAN_POINT ( 'NONE',  ( -136.8705256357208668, -1072.742444906768242, -28.88783501520649821 ) ) ;
#7759=ORIENTED_EDGE ( 'NONE', *, *, #19963, .F. ) ;
#7760=CARTESIAN_POINT ( 'NONE',  ( -135.7895026000614678, -1074.740959209980247, 27.50000000000646239 ) ) ;
#7783=CARTESIAN_POINT ( 'NONE',  ( 146.4450000000001921, -210.0000000000003411, -27.49999999999356604 ) ) ;
#7785=CARTESIAN_POINT ( 'NONE',  ( 123.4701789281961766, -1093.702342252439848, 31.88926668738014669 ) ) ;
#7789=FACE_BOUND ( 'NONE', #7117, .T. ) ;
#7798=CYLINDRICAL_SURFACE ( 'NONE', #13306, 2.500000000000002220 ) ;
#7804=ORIENTED_EDGE ( 'NONE', *, *, #17971, .T. ) ;
#7818=DIRECTION ( 'NONE',  ( 1.000000000000000000, -0.000000000000000000, 6.982962677686266711E-15 ) ) ;
#7828=DIRECTION ( 'NONE',  ( -1.000000000000000000, -2.775557561562891351E-17, 0.000000000000000000 ) ) ;
#7832=ORIENTED_EDGE ( 'NONE', *, *, #18645, .T. ) ;
#7833=ORIENTED_EDGE ( 'NONE', *, *, #1074, .T. ) ;
#7838=AXIS2_PLACEMENT_3D ( 'NONE', #18559, #5649, #12942 ) ;
#7842=CARTESIAN_POINT ( 'NONE',  ( -127.8082730365395179, 87.69306101368195527, 27.50000000000646949 ) ) ;
#7846=ORIENTED_EDGE ( 'NONE', *, *, #11341, .F. ) ;
#7866=APPLICATION_CONTEXT ( 'automotive_design' ) ;
#7875=CARTESIAN_POINT ( 'NONE',  ( -146.0000000000004832, -784.4690652294799520, -27.94499999999356632 ) ) ;
#7896=LINE ( 'NONE', #7525, #20741 ) ;
#7903=CARTESIAN_POINT ( 'NONE',  ( 123.1027542345835002, -1094.184478438182623, 31.11216498479339521 ) ) ;
#7905=EDGE_LOOP ( 'NONE', ( #10697, #6070, #4877, #4690 ) ) ;
#7909=PLANE ( 'NONE',  #7147 ) ;
#7926=ADVANCED_FACE ( 'NONE', ( #20474 ), #12507, .F. ) ;
#7935=ORIENTED_EDGE ( 'NONE', *, *, #3572, .T. ) ;
#7955=ORIENTED_EDGE ( 'NONE', *, *, #20131, .F. ) ;
#7961=CARTESIAN_POINT ( 'NONE',  ( -127.4426065742858043, 88.22361005463049821, 32.37408494914630097 ) ) ;
#7962=ORIENTED_EDGE ( 'NONE', *, *, #6269, .T. ) ;
#7966=AXIS2_PLACEMENT_3D ( 'NONE', #6922, #14536, #18154 ) ;
#7968=ADVANCED_FACE ( 'NONE', ( #902, #4771 ), #6592, .T. ) ;
#7971=EDGE_LOOP ( 'NONE', ( #21664, #7315, #19262, #11771 ) ) ;
#7990=ORIENTED_EDGE ( 'NONE', *, *, #2806, .T. ) ;
#7998=CARTESIAN_POINT ( 'NONE',  ( -194.7500000000000284, -494.4690652294800657, 30.00000000000675726 ) ) ;
#8014=ORIENTED_EDGE ( 'NONE', *, *, #8236, .T. ) ;
#8018=CARTESIAN_POINT ( 'NONE',  ( 131.9719027401102380, 81.29225469460293141, -31.88744336596581519 ) ) ;
#8043=ADVANCED_FACE ( 'NONE', ( #17683 ), #4748, .F. ) ;
#8060=DIRECTION ( 'NONE',  ( 1.000000000000000000, -0.000000000000000000, 6.982962677686266711E-15 ) ) ;
#8066=CIRCLE ( 'NONE', #3792, 2.055000000000001492 ) ;
#8075=ORIENTED_EDGE ( 'NONE', *, *, #14777, .F. ) ;
#8078=LINE ( 'NONE', #4326, #20066 ) ;
#8079=DIRECTION ( 'NONE',  ( -1.000000000000000000, 1.408839003528726857E-14, 6.982962677686266711E-15 ) ) ;
#8085=ORIENTED_EDGE ( 'NONE', *, *, #21208, .F. ) ;
#8089=DIRECTION ( 'NONE',  ( 0.6964005597823107463, -0.7176533009294141507, 6.982962677686266711E-15 ) ) ;
#8106=CONICAL_SURFACE ( 'NONE', #10049, 2.055000000000001492, 0.7853981633974633780 ) ;
#8117=CARTESIAN_POINT ( 'NONE',  ( 171.6502151485116769, 95.33502053007514121, -32.49999999999322853 ) ) ;
#8118=ADVANCED_FACE ( 'NONE', ( #5567 ), #19799, .F. ) ;
#8125=AXIS2_PLACEMENT_3D ( 'NONE', #6011, #7828, #15101 ) ;
#8132=EDGE_CURVE ( 'NONE', #14202, #404, #18624, .T. ) ;
#8146=EDGE_LOOP ( 'NONE', ( #7685, #979 ) ) ;
#8153=FACE_OUTER_BOUND ( 'NONE', #21023, .T. ) ;
#8155=VERTEX_POINT ( 'NONE', #11393 ) ;
#8157=EDGE_CURVE ( 'NONE', #17523, #20328, #37, .T. ) ;
#8165=ORIENTED_EDGE ( 'NONE', *, *, #14060, .F. ) ;
#8187=CARTESIAN_POINT ( 'NONE',  ( 194.7499999999997726, -209.9999999999996874, 27.50000000000675371 ) ) ;
#8188=EDGE_CURVE ( 'NONE', #3982, #21618, #15325, .T. ) ;
#8193=LINE ( 'NONE', #10128, #12742 ) ;
#8195=CYLINDRICAL_SURFACE ( 'NONE', #970, 2.500000000000002220 ) ;
#8206=DIRECTION ( 'NONE',  ( 0.000000000000000000, 0.000000000000000000, -1.000000000000000000 ) ) ;
#8209=ORIENTED_EDGE ( 'NONE', *, *, #22002, .T. ) ;
#8215=ORIENTED_EDGE ( 'NONE', *, *, #279, .T. ) ;
#8219=ORIENTED_EDGE ( 'NONE', *, *, #1512, .F. ) ;
#8236=EDGE_CURVE ( 'NONE', #10799, #2037, #22461, .T. ) ;
#8242=AXIS2_PLACEMENT_3D ( 'NONE', #9557, #20528, #23480 ) ;
#8249=CARTESIAN_POINT ( 'NONE',  ( 146.4450000000002206, -801.0618695410406644, -27.49999999999356604 ) ) ;
#8254=AXIS2_PLACEMENT_3D ( 'NONE', #11088, #18409, #4034 ) ;
#8260=VERTEX_POINT ( 'NONE', #4234 ) ;
#8273=ORIENTED_EDGE ( 'NONE', *, *, #15346, .T. ) ;
#8297=AXIS2_PLACEMENT_3D ( 'NONE', #19271, #2740, #10124 ) ;
#8309=DIRECTION ( 'NONE',  ( -0.7071067811865320296, 9.875400524328840493E-15, 0.7071067811865631159 ) ) ;
#8315=LINE ( 'NONE', #17487, #7313 ) ;
#8321=CARTESIAN_POINT ( 'NONE',  ( -126.9537165176732287, 88.92563123478208809, 31.88926668738024972 ) ) ;
#8323=CARTESIAN_POINT ( 'NONE',  ( -135.0388036711515838, -1076.089031023631605, -31.99040335529160117 ) ) ;
#8333=CONICAL_SURFACE ( 'NONE', #13768, 2.055000000000001492, 0.7853981633974633780 ) ;
#8334=DIRECTION ( 'NONE',  ( -0.000000000000000000, -0.000000000000000000, -1.000000000000000000 ) ) ;
#8335=FACE_OUTER_BOUND ( 'NONE', #18064, .T. ) ;
#8373=ORIENTED_EDGE ( 'NONE', *, *, #14175, .T. ) ;
#8374=EDGE_CURVE ( 'NONE', #15690, #22268, #23185, .T. ) ;
#8382=ORIENTED_EDGE ( 'NONE', *, *, #10080, .F. ) ;
#8392=DIRECTION ( 'NONE',  ( -6.753181414994864868E-15, 6.753181414994864868E-15, -1.000000000000000000 ) ) ;
#8394=EDGE_CURVE ( 'NONE', #12953, #14948, #19545, .T. ) ;
#8402=AXIS2_PLACEMENT_3D ( 'NONE', #23634, #7093, #21819 ) ;
#8419=DIRECTION ( 'NONE',  ( -1.000000000000000000, 1.408839003528726857E-14, 6.982962677686266711E-15 ) ) ;
#8422=LINE ( 'NONE', #5501, #6497 ) ;
#8432=DIRECTION ( 'NONE',  ( 6.753181414994864868E-15, 0.000000000000000000, -1.000000000000000000 ) ) ;
#8448=CARTESIAN_POINT ( 'NONE',  ( -135.4687158836535161, -1075.321440059930637, -32.43450926607474827 ) ) ;
#8454=DIRECTION ( 'NONE',  ( 1.000000000000000000, -0.000000000000000000, -0.000000000000000000 ) ) ;
#8457=CARTESIAN_POINT ( 'NONE',  ( 134.1263161626748968, 77.68610759098272922, -29.83733181946745816 ) ) ;
#8460=VECTOR ( 'NONE', #1107, 1000.000000000000000 ) ;
#8462=DIRECTION ( 'NONE',  ( 1.350636282998972974E-14, 0.000000000000000000, -1.000000000000000000 ) ) ;
#8473=AXIS2_PLACEMENT_3D ( 'NONE', #1255, #21418, #17449 ) ;
#8480=VECTOR ( 'NONE', #19870, 1000.000000000000000 ) ;
#8499=VERTEX_POINT ( 'NONE', #14742 ) ;
#8539=DIRECTION ( 'NONE',  ( -1.000000000000000000, 1.408839003528726857E-14, 6.982962677686266711E-15 ) ) ;
#8552=DIRECTION ( 'NONE',  ( 0.000000000000000000, 0.000000000000000000, 1.000000000000000000 ) ) ;
#8557=CARTESIAN_POINT ( 'NONE',  ( 145.0000000000000284, 0.000000000000000000, 90.00000000000000000 ) ) ;
#8565=FACE_OUTER_BOUND ( 'NONE', #21396, .T. ) ;
#8566=VERTEX_POINT ( 'NONE', #8954 ) ;
#8570=CARTESIAN_POINT ( 'NONE',  ( -134.7157571289271516, -1076.659463591458007, -31.25700618919322693 ) ) ;
#8571=ORIENTED_EDGE ( 'NONE', *, *, #10506, .T. ) ;
#8576=CARTESIAN_POINT ( 'NONE',  ( 133.4121500950862469, 78.90641005980357647, -27.75009929603928072 ) ) ;
#8577=EDGE_CURVE ( 'NONE', #4130, #12774, #12844, .T. ) ;
#8581=CYLINDRICAL_SURFACE ( 'NONE', #6264, 2.500000000000002220 ) ;
#8586=ORIENTED_EDGE ( 'NONE', *, *, #6019, .F. ) ;
#8587=EDGE_CURVE ( 'NONE', #1686, #963, #1790, .T. ) ;
#8593=ORIENTED_EDGE ( 'NONE', *, *, #6926, .T. ) ;
#8594=CARTESIAN_POINT ( 'NONE',  ( -136.9304241666585824, -1072.629629052829841, 30.80845853161013892 ) ) ;
#8640=EDGE_CURVE ( 'NONE', #19464, #17109, #15106, .T. ) ;
#8655=DIRECTION ( 'NONE',  ( 0.000000000000000000, -1.000000000000000000, 0.000000000000000000 ) ) ;
#8660=EDGE_LOOP ( 'NONE', ( #1945, #5773, #7935, #14750 ) ) ;
#8671=VECTOR ( 'NONE', #21185, 1000.000000000000114 ) ;
#8682=ORIENTED_EDGE ( 'NONE', *, *, #415, .T. ) ;
#8686=CARTESIAN_POINT ( 'NONE',  ( -135.7895026000616667, -1074.740959209979792, -27.49999999999351985 ) ) ;
#8689=VERTEX_POINT ( 'NONE', #6267 ) ;
#8694=CARTESIAN_POINT ( 'NONE',  ( 133.6263423143007572, 78.54310546248434832, -28.00764941310470135 ) ) ;
#8705=ADVANCED_FACE ( 'NONE', ( #15470 ), #12276, .F. ) ;
#8718=EDGE_LOOP ( 'NONE', ( #10530, #19645, #10578, #10680 ) ) ;
#8727=CARTESIAN_POINT ( 'NONE',  ( -128.5330911521621431, -1074.345258785412625, 30.00000000000641620 ) ) ;
#8744=EDGE_LOOP ( 'NONE', ( #547, #15983, #16105, #15606 ) ) ;
#8749=ORIENTED_EDGE ( 'NONE', *, *, #16864, .F. ) ;
#8751=CARTESIAN_POINT ( 'NONE',  ( -129.3180659214438890, 85.45079184243574844, -30.32849798811265885 ) ) ;
#8757=ADVANCED_FACE ( 'NONE', ( #11985 ), #12675, .F. ) ;
#8760=CARTESIAN_POINT ( 'NONE',  ( 133.6912351773691228, 78.43256762916516323, 31.88926668738024972 ) ) ;
#8772=CYLINDRICAL_SURFACE ( 'NONE', #17579, 2.500000000000002220 ) ;
#8776=DIRECTION ( 'NONE',  ( 1.000000000000000000, -1.408839003528726857E-14, -6.982962677686266711E-15 ) ) ;
#8788=CARTESIAN_POINT ( 'NONE',  ( 155.0000000000000284, -500.0000000000000000, 30.00000000000001421 ) ) ;
#8790=CARTESIAN_POINT ( 'NONE',  ( 155.0000000000000568, -801.0618695410399823, 30.00000000000648015 ) ) ;
#8797=EDGE_LOOP ( 'NONE', ( #4434, #800 ) ) ;
#8800=CARTESIAN_POINT ( 'NONE',  ( 146.0000000000002274, -210.0000000000003411, -29.99999999999356604 ) ) ;
#8802=FACE_BOUND ( 'NONE', #5929, .T. ) ;
#8814=ORIENTED_EDGE ( 'NONE', *, *, #19198, .F. ) ;
#8837=AXIS2_PLACEMENT_3D ( 'NONE', #3287, #16344, #7041 ) ;
#8840=CIRCLE ( 'NONE', #10008, 2.499999999999998668 ) ;
#8863=VECTOR ( 'NONE', #11578, 1000.000000000000114 ) ;
#8885=CARTESIAN_POINT ( 'NONE',  ( 133.8109447024529004, 78.22816056888504477, 31.65640384616916947 ) ) ;
#8886=AXIS2_PLACEMENT_3D ( 'NONE', #16788, #3969, #22691 ) ;
#8887=AXIS2_PLACEMENT_3D ( 'NONE', #3215, #10627, #828 ) ;
#8896=ADVANCED_FACE ( 'NONE', ( #13043 ), #16503, .F. ) ;
#8909=AXIS2_PLACEMENT_3D ( 'NONE', #7560, #14951, #16745 ) ;
#8912=ORIENTED_EDGE ( 'NONE', *, *, #3122, .T. ) ;
#8925=DIRECTION ( 'NONE',  ( -1.000000000000000000, -2.775557561562891351E-17, 0.000000000000000000 ) ) ;
#8930=DIRECTION ( 'NONE',  ( 1.350636282998972974E-14, 0.000000000000000000, -1.000000000000000000 ) ) ;
#8932=FACE_OUTER_BOUND ( 'NONE', #12438, .T. ) ;
#8934=ADVANCED_FACE ( 'NONE', ( #18544 ), #3466, .F. ) ;
#8950=CARTESIAN_POINT ( 'NONE',  ( -127.0272233253969318, 88.82062435172005621, -28.00764941310471201 ) ) ;
#8954=CARTESIAN_POINT ( 'NONE',  ( -135.7895026000616667, -1074.740959209979792, -27.49999999999351985 ) ) ;
#8956=DIRECTION ( 'NONE',  ( -1.000000000000000000, 1.408839003528726857E-14, 6.982962677686266711E-15 ) ) ;
#8958=ORIENTED_EDGE ( 'NONE', *, *, #14505, .T. ) ;
#8974=DIRECTION ( 'NONE',  ( 1.350636282998972974E-14, 0.000000000000000000, -1.000000000000000000 ) ) ;
#8992=CARTESIAN_POINT ( 'NONE',  ( 155.0000000000000284, -500.0000000000000000, -27.49999999999996803 ) ) ;
#8993=CARTESIAN_POINT ( 'NONE',  ( 132.9250442248334139, 79.72427207779767855, 32.50000000000646594 ) ) ;
#9006=DIRECTION ( 'NONE',  ( 0.000000000000000000, -1.000000000000000000, 0.000000000000000000 ) ) ;
#9033=AXIS2_PLACEMENT_3D ( 'NONE', #9166, #16524, #16412 ) ;
#9035=LINE ( 'NONE', #18202, #10851 ) ;
#9047=CARTESIAN_POINT ( 'NONE',  ( -135.7895026000614109, -1074.740959209980247, 32.50000000000646594 ) ) ;
#9054=CARTESIAN_POINT ( 'NONE',  ( -126.8176664439032919, 89.11954614941136299, -28.34359615383082343 ) ) ;
#9055=AXIS2_PLACEMENT_3D ( 'NONE', #19478, #15429, #2935 ) ;
#9059=DIRECTION ( 'NONE',  ( -1.000000000000000000, 1.408839003528726857E-14, 6.982962677686266711E-15 ) ) ;
#9080=ADVANCED_FACE ( 'NONE', ( #20478 ), #323, .F. ) ;
#9087=ORIENTED_EDGE ( 'NONE', *, *, #1195, .F. ) ;
#9096=CIRCLE ( 'NONE', #6005, 2.055000000000001492 ) ;
#9126=DIRECTION ( 'NONE',  ( 0.000000000000000000, 0.000000000000000000, 1.000000000000000000 ) ) ;
#9127=DIRECTION ( 'NONE',  ( 0.7071067811865416886, 0.000000000000000000, -0.7071067811865532349 ) ) ;
#9136=CARTESIAN_POINT ( 'NONE',  ( 123.5476367174094179, -1093.600214943837500, -28.00764941310472977 ) ) ;
#9140=ADVANCED_FACE ( 'NONE', ( #12081 ), #3377, .F. ) ;
#9149=CARTESIAN_POINT ( 'NONE',  ( -146.0000000000005116, -784.4690652294799520, -29.99999999999356604 ) ) ;
#9151=ORIENTED_EDGE ( 'NONE', *, *, #6248, .F. ) ;
#9157=VERTEX_POINT ( 'NONE', #23124 ) ;
#9160=AXIS2_PLACEMENT_3D ( 'NONE', #6016, #15578, #4450 ) ;
#9162=ORIENTED_EDGE ( 'NONE', *, *, #19795, .F. ) ;
#9164=CARTESIAN_POINT ( 'NONE',  ( -136.5237489982504826, -1073.391313005787879, 28.00660068667239955 ) ) ;
#9166=CARTESIAN_POINT ( 'NONE',  ( 155.0000000000000284, -500.0000000000000000, -29.99999999999997158 ) ) ;
#9172=CARTESIAN_POINT ( 'NONE',  ( -127.8082730365391058, 87.69306101368243844, -32.49999999999352696 ) ) ;
#9174=DIRECTION ( 'NONE',  ( -1.000000000000000000, 0.000000000000000000, 0.000000000000000000 ) ) ;
#9190=ADVANCED_FACE ( 'NONE', ( #6821 ), #15663, .F. ) ;
#9200=AXIS2_PLACEMENT_3D ( 'NONE', #1434, #3137, #3242 ) ;
#9201=FACE_OUTER_BOUND ( 'NONE', #18344, .T. ) ;
#9207=DIRECTION ( 'NONE',  ( 1.350636282998972974E-14, 0.000000000000000000, -1.000000000000000000 ) ) ;
#9215=AXIS2_PLACEMENT_3D ( 'NONE', #14608, #12837, #14735 ) ;
#9218=VECTOR ( 'NONE', #12568, 1000.000000000000000 ) ;
#9228=CONICAL_SURFACE ( 'NONE', #11973, 2.055000000000001492, 0.7853981633974633780 ) ;
#9230=CARTESIAN_POINT ( 'NONE',  ( 125.4586218058189075, -1091.022788359628976, 28.11255663403414928 ) ) ;
#9232=CARTESIAN_POINT ( 'NONE',  ( -127.9021285790841205, 87.55595642181886262, 32.50000000000646594 ) ) ;
#9233=CARTESIAN_POINT ( 'NONE',  ( 134.1261853992450312, 77.68633335585877830, 29.67072815018523713 ) ) ;
#9251=CARTESIAN_POINT ( 'NONE',  ( 146.0000000000002274, -801.0618695410406644, -29.99999999999356604 ) ) ;
#9254=CIRCLE ( 'NONE', #394, 2.499999999999998668 ) ;
#9257=VECTOR ( 'NONE', #11202, 1000.000000000000000 ) ;
#9261=CIRCLE ( 'NONE', #13918, 2.055000000000001492 ) ;
#9267=CARTESIAN_POINT ( 'NONE',  ( 122.9870427404257498, -1094.335589877584880, -30.66034227022087677 ) ) ;
#9279=AXIS2_PLACEMENT_3D ( 'NONE', #23528, #19523, #17969 ) ;
#9285=B_SPLINE_CURVE_WITH_KNOTS ( 'NONE', 3,
 ( #18608, #20300, #9348, #7276, #14787, #7633, #14670, #159, #3414, #5354, #13124, #11183, #5474, #16707, #10828, #12882, #16816, #9464, #11055, #22115, #7403, #9230, #12776, #18375, #275, #16593, #12644, #1608 ),
 .UNSPECIFIED., .F., .F.,
 ( 4, 2, 2, 2, 2, 2, 2, 2, 2, 2, 2, 2, 2, 4 ),
 ( 0.007862850516742021789, 0.008354729399060772249, 0.008846608281379520974, 0.009830366046016477191, 0.01032224492833494489, 0.01081412381065341086, 0.01130600269297188029, 0.01179788157529034626, 0.01278163933992727125, 0.01327351822224584824, 0.01376539710456442522, 0.01425727598688300221, 0.01474915486920157920, 0.01573291263383920502 ),
 .UNSPECIFIED. ) ;
#9289=DIRECTION ( 'NONE',  ( 0.6964005597823107463, -0.7176533009294141507, 6.982962677686266711E-15 ) ) ;
#9296=B_SPLINE_CURVE_WITH_KNOTS ( 'NONE', 3,
 ( #14790, #16120, #12532, #22118, #1835, #5594, #14337, #19849, #19960, #3642, #18046, #14550, #3297, #11058, #9233, #18165, #3418, #18379, #16599, #20453, #1373, #12783, #8885, #8760, #23468, #56, #16250, #23594, #1612, #20089, #8993, #12885 ),
 .UNSPECIFIED., .F., .F.,
 ( 4, 2, 2, 2, 2, 2, 2, 2, 2, 2, 2, 2, 2, 2, 2, 4 ),
 ( 0.000000000000000000, 0.0004914281572963739766, 0.0009828563145927479532, 0.001474284471889121930, 0.001965712629185495906, 0.002457140786481870100, 0.002948568943778243859, 0.003931425258371016099, 0.004422853415667405905, 0.004914281572963798313, 0.005405709730260188986, 0.005897137887556580527, 0.006388566044852972067, 0.006879994202149363608, 0.007371422359445755149, 0.007862850516742146689 ),
 .UNSPECIFIED. ) ;
#9305=CARTESIAN_POINT ( 'NONE',  ( -127.4422799395774888, 88.22408193900511719, -32.37389708099360064 ) ) ;
#9312=DIRECTION ( 'NONE',  ( 0.6964005597823107463, -0.7176533009294141507, 6.982962677686266711E-15 ) ) ;
#9320=CARTESIAN_POINT ( 'NONE',  ( -175.1609685624536326, -1088.719770019218913, 30.00000000000675726 ) ) ;
#9327=CARTESIAN_POINT ( 'NONE',  ( 125.9265396616750223, -1090.374350352354895, -30.65604281379834717 ) ) ;
#9336=ORIENTED_EDGE ( 'NONE', *, *, #8132, .T. ) ;
#9341=CARTESIAN_POINT ( 'NONE',  ( -134.5892462183198290, -1076.881310361372016, 30.65375098132850340 ) ) ;
#9348=CARTESIAN_POINT ( 'NONE',  ( 124.6651547408757210, -1092.106598813447135, 32.48437713430730156 ) ) ;
#9350=CARTESIAN_POINT ( 'NONE',  ( -128.3589811823735545, 86.88495287852394711, 32.37380477188061434 ) ) ;
#9367=FACE_OUTER_BOUND ( 'NONE', #17550, .T. ) ;
#9368=CARTESIAN_POINT ( 'NONE',  ( 155.0000000000000284, -210.0000000000003411, -29.99999999999350564 ) ) ;
#9374=CARTESIAN_POINT ( 'NONE',  ( 145.9999999999997726, -209.9999999999996874, 32.05500000000641592 ) ) ;
#9393=DIRECTION ( 'NONE',  ( 0.000000000000000000, -1.000000000000000000, 0.000000000000000000 ) ) ;
#9394=AXIS2_PLACEMENT_3D ( 'NONE', #14789, #55, #18610 ) ;
#9398=AXIS2_PLACEMENT_3D ( 'NONE', #21553, #19733, #9207 ) ;
#9402=CARTESIAN_POINT ( 'NONE',  ( -136.9530201128892486, -1072.586991580761151, 30.65186413114638952 ) ) ;
#9404=ORIENTED_EDGE ( 'NONE', *, *, #23180, .F. ) ;
#9427=CARTESIAN_POINT ( 'NONE',  ( 155.0000000000000284, -500.0000000000000000, -29.99999999999997158 ) ) ;
#9430=VECTOR ( 'NONE', #6500, 1000.000000000000000 ) ;
#9435=CARTESIAN_POINT ( 'NONE',  ( 145.0000000000000568, -1000.000000000000000, 90.00000000000000000 ) ) ;
#9450=AXIS2_PLACEMENT_3D ( 'NONE', #21276, #23311, #17420 ) ;
#9451=VERTEX_POINT ( 'NONE', #648 ) ;
#9452=EDGE_CURVE ( 'NONE', #471, #5229, #7896, .T. ) ;
#9453=AXIS2_PLACEMENT_3D ( 'NONE', #4905, #4543, #9999 ) ;
#9455=ORIENTED_EDGE ( 'NONE', *, *, #17276, .T. ) ;
#9456=CARTESIAN_POINT ( 'NONE',  ( -146.0000000000005116, -784.4690652294799520, -29.99999999999356604 ) ) ;
#9464=CARTESIAN_POINT ( 'NONE',  ( 125.8137507114124531, -1090.531233726929486, 28.88700448195640647 ) ) ;
#9473=CARTESIAN_POINT ( 'NONE',  ( 0.000000000000000000, 0.000000000000000000, 0.000000000000000000 ) ) ;
#9478=AXIS2_PLACEMENT_3D ( 'NONE', #13346, #4113, #11524 ) ;
#9502=LINE ( 'NONE', #20227, #17322 ) ;
#9528=DIRECTION ( 'NONE',  ( -1.110223024625157172E-14, 0.000000000000000000, -1.000000000000000000 ) ) ;
#9536=CARTESIAN_POINT ( 'NONE',  ( 194.7499999999997158, -209.9999999999996874, 32.50000000000675726 ) ) ;
#9543=DIRECTION ( 'NONE',  ( -0.7232617928448825673, 0.6905739489807055653, 6.982962677686266711E-15 ) ) ;
#9546=CARTESIAN_POINT ( 'NONE',  ( -128.6141261030693670, 86.50721885637456410, -27.81095155082708459 ) ) ;
#9557=CARTESIAN_POINT ( 'NONE',  ( 126.3653543294811499, 77.28387428943223370, 30.00000000000641620 ) ) ;
#9559=VECTOR ( 'NONE', #12678, 1000.000000000000000 ) ;
#9563=CARTESIAN_POINT ( 'NONE',  ( -135.8696211158501228, -1074.595399753385209, -32.49999999999353406 ) ) ;
#9566=CARTESIAN_POINT ( 'NONE',  ( -135.0388036711513564, -1076.089031023632515, 28.00959664470840593 ) ) ;
#9568=AXIS2_PLACEMENT_3D ( 'NONE', #18906, #3925, #4043 ) ;
#9576=ADVANCED_FACE ( 'NONE', ( #4741 ), #19454, .F. ) ;
#9583=CARTESIAN_POINT ( 'NONE',  ( -127.9021285790841205, 87.55595642181887683, 27.50000000000646239 ) ) ;
#9586=CYLINDRICAL_SURFACE ( 'NONE', #20359, 155.0000000000000284 ) ;
#9588=VERTEX_POINT ( 'NONE', #2567 ) ;
#9603=FACE_OUTER_BOUND ( 'NONE', #5783, .T. ) ;
#9604=CARTESIAN_POINT ( 'NONE',  ( 124.4701338314438317, -1092.369831568442805, 32.50000000000646594 ) ) ;
#9610=CARTESIAN_POINT ( 'NONE',  ( 125.6044290879531644, 79.19280534549544370, -29.99999999999356604 ) ) ;
#9625=CARTESIAN_POINT ( 'NONE',  ( -146.4450000000000784, -784.4690652294805204, 30.00000000000641975 ) ) ;
#9628=ADVANCED_FACE ( 'NONE', ( #2911 ), #8106, .F. ) ;
#9629=ORIENTED_EDGE ( 'NONE', *, *, #107, .T. ) ;
#9648=EDGE_LOOP ( 'NONE', ( #16654, #7255 ) ) ;
#9655=UNCERTAINTY_MEASURE_WITH_UNIT (LENGTH_MEASURE( 1.000000000000000082E-05 ), #11540, 'distance_accuracy_value', 'NONE');
#9665=AXIS2_PLACEMENT_3D ( 'NONE', #18055, #12896, #1503 ) ;
#9697=ORIENTED_EDGE ( 'NONE', *, *, #14215, .F. ) ;
#9698=CARTESIAN_POINT ( 'NONE',  ( -136.8330323738933316, -1072.812977866783285, -28.74099766568594205 ) ) ;
#9709=ORIENTED_EDGE ( 'NONE', *, *, #23209, .T. ) ;
#9714=CARTESIAN_POINT ( 'NONE',  ( 119.9257125005557043, -1087.686723660050802, -29.99999999999356248 ) ) ;
#9715=ORIENTED_EDGE ( 'NONE', *, *, #3852, .F. ) ;
#9729=DIRECTION ( 'NONE',  ( 0.000000000000000000, 0.000000000000000000, -1.000000000000000000 ) ) ;
#9730=CARTESIAN_POINT ( 'NONE',  ( 123.2631315123082345, -1093.974511992576709, 31.53022738271477721 ) ) ;
#9744=CARTESIAN_POINT ( 'NONE',  ( 119.6158142514527327, -1087.367367941136308, 30.00000000000641620 ) ) ;
#9748=EDGE_CURVE ( 'NONE', #18892, #14056, #17756, .T. ) ;
#9756=ADVANCED_FACE ( 'NONE', ( #18151 ), #18363, .F. ) ;
#9760=CARTESIAN_POINT ( 'NONE',  ( 124.4701338314438317, -1092.369831568442805, 32.50000000000646594 ) ) ;
#9774=DIRECTION ( 'NONE',  ( -0.7071067811865320296, 9.875400524328840493E-15, 0.7071067811865631159 ) ) ;
#9785=VERTEX_POINT ( 'NONE', #21760 ) ;
#9812=VECTOR ( 'NONE', #14362, 999.9999999999998863 ) ;
#9814=CARTESIAN_POINT ( 'NONE',  ( -134.8087563975452667, -1076.495802945234345, 31.53271418707683793 ) ) ;
#9816=EDGE_LOOP ( 'NONE', ( #18568, #16887, #17535, #2816 ) ) ;
#9841=CARTESIAN_POINT ( 'NONE',  ( 131.7935180829131809, 81.58110848117762259, -28.46728581292316917 ) ) ;
#9845=APPLICATION_CONTEXT ( 'automotive_design' ) ;
#9849=CARTESIAN_POINT ( 'NONE',  ( 124.3711180590063634, -1092.503257236081254, 27.50000000000645528 ) ) ;
#9854=ORIENTED_EDGE ( 'NONE', *, *, #4146, .T. ) ;
#9863=CARTESIAN_POINT ( 'NONE',  ( 119.6158142514527185, -1087.367367941136308, 32.05500000000641592 ) ) ;
#9869=VERTEX_POINT ( 'NONE', #18833 ) ;
#9873=ORIENTED_EDGE ( 'NONE', *, *, #11595, .T. ) ;
#9879=EDGE_LOOP ( 'NONE', ( #9917, #4180, #7013, #6931 ) ) ;
#9886=EDGE_CURVE ( 'NONE', #22288, #8566, #3931, .T. ) ;
#9892=EDGE_LOOP ( 'NONE', ( #11751, #860 ) ) ;
#9898=EDGE_CURVE ( 'NONE', #16414, #15690, #16926, .T. ) ;
#9909=CARTESIAN_POINT ( 'NONE',  ( -146.0000000000005684, -206.5240652294800725, -29.99999999999356604 ) ) ;
#9917=ORIENTED_EDGE ( 'NONE', *, *, #17971, .F. ) ;
#9920=ADVANCED_FACE ( 'NONE', ( #4809 ), #12220, .F. ) ;
#9924=CARTESIAN_POINT ( 'NONE',  ( 145.9999999999998295, -209.9999999999996874, 27.94500000000641649 ) ) ;
#9934=FACE_BOUND ( 'NONE', #9892, .T. ) ;
#9936=ORIENTED_EDGE ( 'NONE', *, *, #18314, .T. ) ;
#9949=CARTESIAN_POINT ( 'NONE',  ( -158.1195828810602109, 116.4077317428687479, -27.49999999999322498 ) ) ;
#9952=DIRECTION ( 'NONE',  ( 5.551115123125785858E-15, 0.000000000000000000, -1.000000000000000000 ) ) ;
#9955=SURFACE_STYLE_FILL_AREA ( #22958 ) ;
#9961=ADVANCED_FACE ( 'NONE', ( #12468 ), #6178, .F. ) ;
#9963=DIRECTION ( 'NONE',  ( 1.000000000000000000, -0.000000000000000000, 6.982962677686266711E-15 ) ) ;
#9971=CARTESIAN_POINT ( 'NONE',  ( 123.9851406373745704, -1093.019934698474117, 27.62610291900636739 ) ) ;
#9978=VERTEX_POINT ( 'NONE', #19657 ) ;
#9990=CARTESIAN_POINT ( 'NONE',  ( 0.000000000000000000, -1000.000000000000000, 90.00000000000000000 ) ) ;
#9994=CARTESIAN_POINT ( 'NONE',  ( -146.0000000000005116, -784.4690652294799520, -29.99999999999356604 ) ) ;
#9999=DIRECTION ( 'NONE',  ( -5.551115123125785858E-15, 5.551115123125785858E-15, -1.000000000000000000 ) ) ;
#10003=AXIS2_PLACEMENT_3D ( 'NONE', #23633, #22053, #10879 ) ;
#10004=CARTESIAN_POINT ( 'NONE',  ( 131.5507733270949586, 81.97201125882446604, 29.34395718620175586 ) ) ;
#10008=AXIS2_PLACEMENT_3D ( 'NONE', #10558, #12397, #14178 ) ;
#10022=EDGE_LOOP ( 'NONE', ( #6641, #8814, #8014, #14147 ) ) ;
#10030=CARTESIAN_POINT ( 'NONE',  ( -129.2206655591605511, -1072.408698320350595, 30.00000000000641620 ) ) ;
#10033=VERTEX_POINT ( 'NONE', #4359 ) ;
#10041=ORIENTED_EDGE ( 'NONE', *, *, #11891, .T. ) ;
#10049=AXIS2_PLACEMENT_3D ( 'NONE', #10311, #17655, #12270 ) ;
#10057=DIRECTION ( 'NONE',  ( 1.110223024625157172E-14, 0.000000000000000000, -1.000000000000000000 ) ) ;
#10064=CIRCLE ( 'NONE', #21237, 145.0000000000000284 ) ;
#10065=VECTOR ( 'NONE', #11587, 1000.000000000000114 ) ;
#10074=ADVANCED_FACE ( 'NONE', ( #2003 ), #1561, .F. ) ;
#10076=CARTESIAN_POINT ( 'NONE',  ( 145.9999999999998295, -209.9999999999996874, 27.94500000000641649 ) ) ;
#10080=EDGE_CURVE ( 'NONE', #10962, #13026, #22285, .T. ) ;
#10085=CARTESIAN_POINT ( 'NONE',  ( -129.2206655591605511, -1072.408698320350595, 30.00000000000641620 ) ) ;
#10087=VERTEX_POINT ( 'NONE', #12823 ) ;
#10088=DIRECTION ( 'NONE',  ( -1.000000000000000000, 1.408839003528726857E-14, 6.982962677686266711E-15 ) ) ;
#10097=ORIENTED_EDGE ( 'NONE', *, *, #7296, .T. ) ;
#10115=DIRECTION ( 'NONE',  ( -1.000000000000000000, 1.408839003528726857E-14, 6.982962677686266711E-15 ) ) ;
#10123=CARTESIAN_POINT ( 'NONE',  ( -158.1195828810602109, 116.4077317428687621, -29.99999999999322498 ) ) ;
#10124=DIRECTION ( 'NONE',  ( -1.110223024625155594E-14, 0.000000000000000000, -1.000000000000000000 ) ) ;
#10128=CARTESIAN_POINT ( 'NONE',  ( 155.0000000000000284, -500.0000000000000000, 27.50000000000001066 ) ) ;
#10131=DIRECTION ( 'NONE',  ( -0.000000000000000000, -1.000000000000000000, -0.000000000000000000 ) ) ;
#10132=EDGE_CURVE ( 'NONE', #885, #19341, #9035, .T. ) ;
#10138=DIRECTION ( 'NONE',  ( -1.000000000000000000, 1.408839003528726857E-14, 6.982962677686266711E-15 ) ) ;
#10156=CARTESIAN_POINT ( 'NONE',  ( 0.000000000000000000, 0.000000000000000000, -90.00000000000000000 ) ) ;
#10161=FACE_OUTER_BOUND ( 'NONE', #10432, .T. ) ;
#10170=DIRECTION ( 'NONE',  ( 1.000000000000000000, 0.000000000000000000, -0.000000000000000000 ) ) ;
#10172=CIRCLE ( 'NONE', #181, 2.055000000000001492 ) ;
#10175=VECTOR ( 'NONE', #22725, 1000.000000000000114 ) ;
#10182=ADVANCED_FACE ( 'NONE', ( #8932 ), #15015, .F. ) ;
#10185=DIRECTION ( 'NONE',  ( 0.6964005597823107463, -0.7176533009294141507, 6.982962677686266711E-15 ) ) ;
#10200=CARTESIAN_POINT ( 'NONE',  ( -146.0000000000000853, -784.4690652294805204, 30.00000000000641620 ) ) ;
#10208=DIRECTION ( 'NONE',  ( 1.110223024625157172E-14, 0.000000000000000000, -1.000000000000000000 ) ) ;
#10219=CARTESIAN_POINT ( 'NONE',  ( 145.0000000000000568, -1000.000000000000000, 90.00000000000000000 ) ) ;
#10224=ORIENTED_EDGE ( 'NONE', *, *, #14365, .F. ) ;
#10249=CARTESIAN_POINT ( 'NONE',  ( -155.0000000000000284, 0.000000000000000000, 90.00000000000000000 ) ) ;
#10266=ORIENTED_EDGE ( 'NONE', *, *, #14978, .F. ) ;
#10268=CARTESIAN_POINT ( 'NONE',  ( -126.5033273815586199, 89.56511165728051083, 30.65186413114638242 ) ) ;
#10296=CARTESIAN_POINT ( 'NONE',  ( -155.0000000000000284, -204.4690652294806057, 30.00000000000648015 ) ) ;
#10307=AXIS2_PLACEMENT_3D ( 'NONE', #15113, #18573, #11489 ) ;
#10311=CARTESIAN_POINT ( 'NONE',  ( -129.2206655591605511, -1072.408698320350595, 30.00000000000641620 ) ) ;
#10312=CARTESIAN_POINT ( 'NONE',  ( 132.1836189744869898, 80.94757571328915446, -32.17188107257626228 ) ) ;
#10334=ORIENTED_EDGE ( 'NONE', *, *, #19326, .T. ) ;
#10337=DIRECTION ( 'NONE',  ( -0.6663528160695909586, -0.2365880903936287138, 0.7071067811865631159 ) ) ;
#10339=CARTESIAN_POINT ( 'NONE',  ( -194.7500000000000568, -204.4690652294800657, 27.50000000000675371 ) ) ;
#10346=AXIS2_PLACEMENT_3D ( 'NONE', #15639, #10459, #2708 ) ;
#10350=CIRCLE ( 'NONE', #12310, 2.055000000000001492 ) ;
#10355=ADVANCED_FACE ( 'NONE', ( #6470 ), #6825, .F. ) ;
#10363=LINE ( 'NONE', #17711, #19107 ) ;
#10373=LINE ( 'NONE', #16277, #17287 ) ;
#10376=DIRECTION ( 'NONE',  ( 1.350636282998972974E-14, 0.000000000000000000, -1.000000000000000000 ) ) ;
#10383=DIRECTION ( 'NONE',  ( 1.000000000000000000, 0.000000000000000000, -0.000000000000000000 ) ) ;
#10395=CARTESIAN_POINT ( 'NONE',  ( -134.8087563975455225, -1076.495802945233663, -28.46728581292316207 ) ) ;
#10402=CARTESIAN_POINT ( 'NONE',  ( 133.9969223633123079, 77.90910650221316303, -28.88783501520648400 ) ) ;
#10423=AXIS2_PLACEMENT_3D ( 'NONE', #23346, #13631, #13859 ) ;
#10426=CIRCLE ( 'NONE', #17729, 2.500000000000002220 ) ;
#10428=AXIS2_PLACEMENT_3D ( 'NONE', #19440, #4618, #4729 ) ;
#10430=AXIS2_PLACEMENT_3D ( 'NONE', #3661, #5260, #19979 ) ;
#10432=EDGE_LOOP ( 'NONE', ( #190, #10097, #21757, #14535 ) ) ;
#10434=CARTESIAN_POINT ( 'NONE',  ( -136.7455495141628887, -1072.977142426287401, 28.46749050845390983 ) ) ;
#10439=DIRECTION ( 'NONE',  ( -5.551115123125785858E-15, 5.551115123125785858E-15, -1.000000000000000000 ) ) ;
#10443=VERTEX_POINT ( 'NONE', #17940 ) ;
#10448=CIRCLE ( 'NONE', #8125, 2.499999999999946709 ) ;
#10457=DIRECTION ( 'NONE',  ( -1.350636282998972974E-14, 0.000000000000000000, -1.000000000000000000 ) ) ;
#10459=DIRECTION ( 'NONE',  ( 0.9289202219288174023, 0.3702799228849934510, 6.982962677686266711E-15 ) ) ;
#10462=DIRECTION ( 'NONE',  ( 1.000000000000000000, -0.000000000000000000, 6.982962677686266711E-15 ) ) ;
#10466=EDGE_LOOP ( 'NONE', ( #9336, #10865 ) ) ;
#10468=ORIENTED_EDGE ( 'NONE', *, *, #14644, .F. ) ;
#10477=DIRECTION ( 'NONE',  ( -1.000000000000000000, 1.408839003528726857E-14, 6.982962677686266711E-15 ) ) ;
#10488=LINE ( 'NONE', #12086, #2635 ) ;
#10491=CARTESIAN_POINT ( 'NONE',  ( 132.8404720734530144, 79.86494211668949106, 27.50000000000646239 ) ) ;
#10496=DIRECTION ( 'NONE',  ( -1.110223024625155594E-14, 0.000000000000000000, -1.000000000000000000 ) ) ;
#10506=EDGE_CURVE ( 'NONE', #21618, #846, #4778, .T. ) ;
#10521=EDGE_CURVE ( 'NONE', #3131, #22831, #14450, .T. ) ;
#10530=ORIENTED_EDGE ( 'NONE', *, *, #19418, .F. ) ;
#10531=CARTESIAN_POINT ( 'NONE',  ( 133.0100681275902730, 79.58233248384551928, -32.48402282453940870 ) ) ;
#10538=EDGE_CURVE ( 'NONE', #6623, #2188, #6541, .T. ) ;
#10558=CARTESIAN_POINT ( 'NONE',  ( 146.4450000000002490, -801.0618695410406644, -29.99999999999356248 ) ) ;
#10560=CARTESIAN_POINT ( 'NONE',  ( -146.4450000000000784, -204.4690652294807194, 30.00000000000641975 ) ) ;
#10568=EDGE_CURVE ( 'NONE', #19646, #6763, #1731, .T. ) ;
#10569=EDGE_LOOP ( 'NONE', ( #18360, #12582, #1898, #23552 ) ) ;
#10574=VERTEX_POINT ( 'NONE', #1978 ) ;
#10578=ORIENTED_EDGE ( 'NONE', *, *, #5363, .T. ) ;
#10581=CARTESIAN_POINT ( 'NONE',  ( -128.2758413234845705, 87.00805048166530753, -32.43450926607476958 ) ) ;
#10587=AXIS2_PLACEMENT_3D ( 'NONE', #19784, #18106, #16183 ) ;
#10589=AXIS2_PLACEMENT_3D ( 'NONE', #2294, #4919, #10376 ) ;
#10597=ORIENTED_EDGE ( 'NONE', *, *, #21478, .F. ) ;
#10608=DIRECTION ( 'NONE',  ( 1.350636282998972974E-14, 0.000000000000000000, -1.000000000000000000 ) ) ;
#10611=LINE ( 'NONE', #6838, #15781 ) ;
#10615=B_SPLINE_CURVE_WITH_KNOTS ( 'NONE', 3,
 ( #11928, #9849, #22753, #13260, #9971, #6087, #6218, #17445, #11685, #17207, #20825, #5852, #5968, #13377, #17084, #13624, #15530, #4020, #21057, #7903, #19238, #9730, #7656, #7785, #20567, #11434, #13508, #2212, #4282, #18994, #2457, #9604 ),
 .UNSPECIFIED., .F., .F.,
 ( 4, 2, 2, 2, 2, 2, 2, 2, 2, 2, 2, 2, 2, 2, 2, 4 ),
 ( 1.430489624538199204E-17, 0.0004914281572963898059, 0.0009828563145927653004, 0.001474284471889140795, 0.001965712629185516289, 0.002457140786481891784, 0.002948568943778267278, 0.003931425258371017833, 0.004422853415667393762, 0.004914281572963768822, 0.005405709730260143883, 0.005897137887556519811, 0.006388566044852895739, 0.006879994202149270800, 0.007371422359445645861, 0.007862850516742021789 ),
 .UNSPECIFIED. ) ;
#10623=EDGE_LOOP ( 'NONE', ( #11410, #20898 ) ) ;
#10627=DIRECTION ( 'NONE',  ( 1.000000000000000000, -0.000000000000000000, -0.000000000000000000 ) ) ;
#10631=FACE_BOUND ( 'NONE', #17485, .T. ) ;
#10648=CARTESIAN_POINT ( 'NONE',  ( 133.4872637682709069, 78.77924338078965150, -27.82770220384453097 ) ) ;
#10649=CIRCLE ( 'NONE', #17551, 2.500000000000002220 ) ;
#10674=CARTESIAN_POINT ( 'NONE',  ( -155.0000000000000284, -204.4690652294806057, 30.00000000000648015 ) ) ;
#10680=ORIENTED_EDGE ( 'NONE', *, *, #9898, .F. ) ;
#10681=CARTESIAN_POINT ( 'NONE',  ( 153.5653415408401941, -1122.352966361446079, -29.99999999999322498 ) ) ;
#10687=CARTESIAN_POINT ( 'NONE',  ( 145.9999999999998010, -209.9999999999996874, 30.00000000000641620 ) ) ;
#10692=ORIENTED_EDGE ( 'NONE', *, *, #12548, .F. ) ;
#10694=ORIENTED_EDGE ( 'NONE', *, *, #2838, .F. ) ;
#10697=ORIENTED_EDGE ( 'NONE', *, *, #279, .F. ) ;
#10722=CARTESIAN_POINT ( 'NONE',  ( 132.8404720734533555, 79.86494211668886578, -32.49999999999351985 ) ) ;
#10733=DIRECTION ( 'NONE',  ( 0.000000000000000000, 0.000000000000000000, -1.000000000000000000 ) ) ;
#10735=CARTESIAN_POINT ( 'NONE',  ( -122.8605704798721945, 82.74225173005939382, -29.99999999999356604 ) ) ;
#10743=ORIENTED_EDGE ( 'NONE', *, *, #1633, .F. ) ;
#10756=AXIS2_PLACEMENT_3D ( 'NONE', #16035, #8552, #23512 ) ;
#10757=CIRCLE ( 'NONE', #7249, 2.499999999999998668 ) ;
#10761=ORIENTED_EDGE ( 'NONE', *, *, #14434, .T. ) ;
#10776=AXIS2_PLACEMENT_3D ( 'NONE', #15715, #13937, #8462 ) ;
#10797=CARTESIAN_POINT ( 'NONE',  ( 125.5946212300928266, -1090.835042168281461, -28.33934113061012283 ) ) ;
#10798=PLANE ( 'NONE',  #21153 ) ;
#10799=VERTEX_POINT ( 'NONE', #15878 ) ;
#10828=CARTESIAN_POINT ( 'NONE',  ( 125.9649699199276967, -1090.320686186013290, 30.16873261443294041 ) ) ;
#10832=CARTESIAN_POINT ( 'NONE',  ( -146.0000000000005400, -784.4690652294799520, -32.05499999999356930 ) ) ;
#10833=MECHANICAL_DESIGN_GEOMETRIC_PRESENTATION_REPRESENTATION('',(#1542),#18126);
#10849=CARTESIAN_POINT ( 'NONE',  ( 155.0000000000000284, -500.0000000000000000, 32.50000000000001421 ) ) ;
#10851=VECTOR ( 'NONE', #23745, 1000.000000000000000 ) ;
#10853=DIRECTION ( 'NONE',  ( -1.000000000000000000, -2.775557561562891351E-17, 0.000000000000000000 ) ) ;
#10860=CARTESIAN_POINT ( 'NONE',  ( 194.7500000000001705, -801.0618695410406644, -27.49999999999322498 ) ) ;
#10865=ORIENTED_EDGE ( 'NONE', *, *, #14355, .T. ) ;
#10867=CARTESIAN_POINT ( 'NONE',  ( 123.1027542345830739, -1094.184478438182850, -28.88783501520646269 ) ) ;
#10872=FACE_BOUND ( 'NONE', #8146, .T. ) ;
#10879=DIRECTION ( 'NONE',  ( 0.000000000000000000, 0.000000000000000000, -1.000000000000000000 ) ) ;
#10880=CYLINDRICAL_SURFACE ( 'NONE', #15707, 2.500000000000002220 ) ;
#10881=ORIENTED_EDGE ( 'NONE', *, *, #4146, .F. ) ;
#10883=DIRECTION ( 'NONE',  ( 0.6964005597823107463, -0.7176533009294141507, 6.982962677686266711E-15 ) ) ;
#10891=CARTESIAN_POINT ( 'NONE',  ( -135.8686487629346402, -1074.597166325825810, 32.50000000000645883 ) ) ;
#10897=CARTESIAN_POINT ( 'NONE',  ( -126.8186628169058139, 89.11812652456539752, -31.65816015360259428 ) ) ;
#10900=B_SPLINE_CURVE_WITH_KNOTS ( 'NONE', 3,
 ( #15975, #4408, #23319, #21510, #14878, #11032, #5451, #10797, #3384, #22211, #5563, #16792, #16563, #21989, #18588, #12973, #9327, #23673, #16681, #10917, #11279, #1937, #18140, #20280, #22092, #12861, #1588, #13096 ),
 .UNSPECIFIED., .F., .F.,
 ( 4, 2, 2, 2, 2, 2, 2, 2, 2, 2, 2, 2, 2, 4 ),
 ( 0.007862850516742106791, 0.008354729399060536327, 0.008846608281378965863, 0.009830366046016317597, 0.01032224492833499346, 0.01081412381065366933, 0.01130600269297234520, 0.01179788157529102106, 0.01278163933992838147, 0.01327351822224696887, 0.01376539710456555453, 0.01425727598688414019, 0.01474915486920272412, 0.01573291263383936808 ),
 .UNSPECIFIED. ) ;
#10917=CARTESIAN_POINT ( 'NONE',  ( 125.6594390352173463, -1090.745324718712482, -31.52881987646419404 ) ) ;
#10935=DIRECTION ( 'NONE',  ( 6.753181414994864868E-15, 0.000000000000000000, -1.000000000000000000 ) ) ;
#10941=CARTESIAN_POINT ( 'NONE',  ( -128.6141261030697649, 86.50721885637406672, 32.18904844917290831 ) ) ;
#10942=ADVANCED_FACE ( 'NONE', ( #22392 ), #21196, .F. ) ;
#10960=CARTESIAN_POINT ( 'NONE',  ( 0.000000000000000000, 0.000000000000000000, 90.00000000000000000 ) ) ;
#10962=VERTEX_POINT ( 'NONE', #22144 ) ;
#10971=VERTEX_POINT ( 'NONE', #3785 ) ;
#10973=CARTESIAN_POINT ( 'NONE',  ( 123.9851406373740446, -1093.019934698474344, -32.37389708099357932 ) ) ;
#10975=CARTESIAN_POINT ( 'NONE',  ( 146.4450000000002490, -210.0000000000003411, -32.49999999999356248 ) ) ;
#10993=CARTESIAN_POINT ( 'NONE',  ( 119.6158142514525480, -1087.367367941136990, -27.94499999999356987 ) ) ;
#11000=CARTESIAN_POINT ( 'NONE',  ( -155.0000000000000284, -494.4690652294799520, -29.99999999999350564 ) ) ;
#11001=CARTESIAN_POINT ( 'NONE',  ( -136.5850230665614902, -1073.277182683704496, 31.88926668738024262 ) ) ;
#11031=CARTESIAN_POINT ( 'NONE',  ( -158.1195828810602109, 116.4077317428687621, -29.99999999999322498 ) ) ;
#11032=CARTESIAN_POINT ( 'NONE',  ( 125.2216071840745997, -1091.349008980712597, -27.81095155082704906 ) ) ;
#11035=DIRECTION ( 'NONE',  ( 0.6964005597823107463, -0.7176533009294141507, 6.982962677686266711E-15 ) ) ;
#11055=CARTESIAN_POINT ( 'NONE',  ( 125.7677891478060417, -1090.595098045220539, 28.74299381080691873 ) ) ;
#11057=CARTESIAN_POINT ( 'NONE',  ( -129.3180659214442301, 85.45079184243522263, 29.67150201188731984 ) ) ;
#11058=CARTESIAN_POINT ( 'NONE',  ( 134.0925202534283756, 77.74453171555596498, 29.33965772977898467 ) ) ;
#11061=LINE ( 'NONE', #18516, #5364 ) ;
#11070=EDGE_CURVE ( 'NONE', #16653, #3521, #4018, .T. ) ;
#11086=CARTESIAN_POINT ( 'NONE',  ( 124.0796955067752521, -1092.893784429268635, -27.57920702976965543 ) ) ;
#11088=CARTESIAN_POINT ( 'NONE',  ( 194.7500000000001990, -801.0618695410406644, -29.99999999999322498 ) ) ;
#11094=VERTEX_POINT ( 'NONE', #11931 ) ;
#11100=EDGE_CURVE ( 'NONE', #20023, #17062, #15646, .T. ) ;
#11111=AXIS2_PLACEMENT_3D ( 'NONE', #3951, #11364, #8206 ) ;
#11112=ADVANCED_FACE ( 'NONE', ( #886 ), #946, .F. ) ;
#11117=CARTESIAN_POINT ( 'NONE',  ( -136.9597779064867780, -1072.574344195404137, 29.33965772977902731 ) ) ;
#11125=CARTESIAN_POINT ( 'NONE',  ( -127.1840658299259417, 88.59589253999689618, -27.82770220384454518 ) ) ;
#11127=FACE_BOUND ( 'NONE', #17862, .T. ) ;
#11129=CARTESIAN_POINT ( 'NONE',  ( -146.0000000000005400, -494.4690652294800657, -32.05499999999356930 ) ) ;
#11145=CARTESIAN_POINT ( 'NONE',  ( -127.9021285790837510, 87.55595642181941685, -32.49999999999351985 ) ) ;
#11149=AXIS2_PLACEMENT_3D ( 'NONE', #10085, #23201, #11783 ) ;
#11163=CARTESIAN_POINT ( 'NONE',  ( -136.1785371930675410, -1074.029921987504395, -27.62591505085369903 ) ) ;
#11166=AXIS2_PLACEMENT_3D ( 'NONE', #3945, #13416, #18792 ) ;
#11167=CARTESIAN_POINT ( 'NONE',  ( -135.7102838464026036, -1074.884883977198115, 32.50000000000647304 ) ) ;
#11183=CARTESIAN_POINT ( 'NONE',  ( 125.8877979345646736, -1090.428239381491267, 30.81384172145508771 ) ) ;
#11185=CYLINDRICAL_SURFACE ( 'NONE', #9394, 2.500000000000002220 ) ;
#11188=CONICAL_SURFACE ( 'NONE', #23495, 2.055000000000001492, 0.7853981633974633780 ) ;
#11202=DIRECTION ( 'NONE',  ( -0.5114233182937452105, 0.4883095222350190001, 0.7071067811865631159 ) ) ;
#11210=AXIS2_PLACEMENT_3D ( 'NONE', #9473, #14914, #3769 ) ;
#11224=CARTESIAN_POINT ( 'NONE',  ( 194.7499999999997442, -801.0618695410399823, 30.00000000000675726 ) ) ;
#11232=CARTESIAN_POINT ( 'NONE',  ( 146.0000000000002274, -801.0618695410406644, -29.99999999999356604 ) ) ;
#11248=CARTESIAN_POINT ( 'NONE',  ( 124.2727838502222966, -1092.635313011623566, -27.51610016701187789 ) ) ;
#11264=VERTEX_POINT ( 'NONE', #11145 ) ;
#11279=CARTESIAN_POINT ( 'NONE',  ( 125.5963796794996341, -1090.832610870657163, -31.65735141704666233 ) ) ;
#11304=FACE_OUTER_BOUND ( 'NONE', #3335, .T. ) ;
#11320=CYLINDRICAL_SURFACE ( 'NONE', #11781, 2.500000000000002220 ) ;
#11323=ORIENTED_EDGE ( 'NONE', *, *, #15028, .F. ) ;
#11326=FACE_OUTER_BOUND ( 'NONE', #14890, .T. ) ;
#11328=ORIENTED_EDGE ( 'NONE', *, *, #20821, .T. ) ;
#11333=DIRECTION ( 'NONE',  ( 0.000000000000000000, 0.000000000000000000, -1.000000000000000000 ) ) ;
#11341=EDGE_CURVE ( 'NONE', #19646, #19464, #10172, .T. ) ;
#11364=DIRECTION ( 'NONE',  ( -0.9423651898111408132, -0.3345860861306287348, 6.982962677686266711E-15 ) ) ;
#11374=ADVANCED_FACE ( 'NONE', ( #13214 ), #13319, .F. ) ;
#11379=CARTESIAN_POINT ( 'NONE',  ( -122.8605704798721945, 82.74225173005939382, -29.99999999999356604 ) ) ;
#11382=CARTESIAN_POINT ( 'NONE',  ( -128.9689330775208020, 85.97690438148627834, -31.65735141704659128 ) ) ;
#11389=CARTESIAN_POINT ( 'NONE',  ( 132.8404720734530144, 79.86494211668949106, 27.50000000000646239 ) ) ;
#11391=CIRCLE ( 'NONE', #178, 2.055000000000001492 ) ;
#11393=CARTESIAN_POINT ( 'NONE',  ( -146.4450000000005048, -494.4690652294800088, -27.49999999999356604 ) ) ;
#11398=DIRECTION ( 'NONE',  ( 1.000000000000000000, -0.000000000000000000, 6.982962677686266711E-15 ) ) ;
#11400=CIRCLE ( 'NONE', #9453, 2.499999999999998668 ) ;
#11401=CARTESIAN_POINT ( 'NONE',  ( -134.5810953439728053, -1076.895678479288563, 29.34395718620174165 ) ) ;
#11404=FACE_OUTER_BOUND ( 'NONE', #22074, .T. ) ;
#11410=ORIENTED_EDGE ( 'NONE', *, *, #4096, .T. ) ;
#11418=CARTESIAN_POINT ( 'NONE',  ( -128.6132171834567544, 86.50814704276137945, 27.82811892742373416 ) ) ;
#11421=FACE_BOUND ( 'NONE', #2385, .T. ) ;
#11423=ORIENTED_EDGE ( 'NONE', *, *, #14505, .F. ) ;
#11425=PRESENTATION_STYLE_ASSIGNMENT (( #4009 ) ) ;
#11434=CARTESIAN_POINT ( 'NONE',  ( 123.7129353098591480, -1093.381627813013665, 32.17229779615543350 ) ) ;
#11453=VERTEX_POINT ( 'NONE', #22686 ) ;
#11461=AXIS2_PLACEMENT_3D ( 'NONE', #6682, #9963, #17660 ) ;
#11463=ORIENTED_EDGE ( 'NONE', *, *, #2348, .F. ) ;
#11482=EDGE_LOOP ( 'NONE', ( #23267, #4564 ) ) ;
#11489=DIRECTION ( 'NONE',  ( 6.982962677686266711E-15, -9.837870180509810443E-29, 1.000000000000000000 ) ) ;
#11499=ORIENTED_EDGE ( 'NONE', *, *, #19348, .T. ) ;
#11500=DIRECTION ( 'NONE',  ( 1.110223024625157172E-14, 0.000000000000000000, -1.000000000000000000 ) ) ;
#11517=ORIENTED_EDGE ( 'NONE', *, *, #15916, .T. ) ;
#11521=CARTESIAN_POINT ( 'NONE',  ( -134.7167544493337914, -1076.657711551589728, 31.26048023074365290 ) ) ;
#11524=DIRECTION ( 'NONE',  ( 1.350636282998972974E-14, 0.000000000000000000, -1.000000000000000000 ) ) ;
#11536=DIRECTION ( 'NONE',  ( -1.350636282998972974E-14, 0.000000000000000000, -1.000000000000000000 ) ) ;
#11540=( LENGTH_UNIT ( ) NAMED_UNIT ( * ) SI_UNIT ( .MILLI., .METRE. ) );
#11541=EDGE_CURVE ( 'NONE', #20119, #10574, #15706, .T. ) ;
#11543=ORIENTED_EDGE ( 'NONE', *, *, #23711, .T. ) ;
#11548=DIRECTION ( 'NONE',  ( 0.4924295582441687857, -0.5074575156280874966, 0.7071067811865630048 ) ) ;
#11555=PRODUCT_DEFINITION ( 'UNKNOWN', '', #19665, #2271 ) ;
#11563=ORIENTED_EDGE ( 'NONE', *, *, #21180, .T. ) ;
#11571=AXIS2_PLACEMENT_3D ( 'NONE', #8790, #12458, #3674 ) ;
#11578=DIRECTION ( 'NONE',  ( 0.7071067811865416886, 0.000000000000000000, -0.7071067811865532349 ) ) ;
#11582=CARTESIAN_POINT ( 'NONE',  ( 145.9999999999997726, -801.0618695410399823, 32.05500000000641592 ) ) ;
#11587=DIRECTION ( 'NONE',  ( -0.5114233182937522049, 0.4883095222350258280, -0.7071067811865532349 ) ) ;
#11591=CARTESIAN_POINT ( 'NONE',  ( -155.0000000000000284, -494.4690652294806910, 32.50000000000648015 ) ) ;
#11595=EDGE_CURVE ( 'NONE', #9869, #1268, #20968, .T. ) ;
#11596=AXIS2_PLACEMENT_3D ( 'NONE', #2828, #22516, #15305 ) ;
#11611=ORIENTED_EDGE ( 'NONE', *, *, #21631, .T. ) ;
#11616=MECHANICAL_DESIGN_GEOMETRIC_PRESENTATION_REPRESENTATION('',(#21973),#4238);
#11618=CIRCLE ( 'NONE', #14674, 2.500000000000002220 ) ;
#11619=DIRECTION ( 'NONE',  ( -1.110223024625157172E-14, 0.000000000000000000, -1.000000000000000000 ) ) ;
#11634=ORIENTED_EDGE ( 'NONE', *, *, #11891, .F. ) ;
#11636=AXIS2_PLACEMENT_3D ( 'NONE', #22796, #10138, #22899 ) ;
#11647=CARTESIAN_POINT ( 'NONE',  ( 155.0000000000000284, -500.0000000000000000, 30.00000000000001421 ) ) ;
#11653=CARTESIAN_POINT ( 'NONE',  ( -136.6960319176259588, -1073.069888270694719, -31.65816015360259428 ) ) ;
#11654=DIRECTION ( 'NONE',  ( 1.000000000000000000, 0.000000000000000000, -0.000000000000000000 ) ) ;
#11666=ORIENTED_EDGE ( 'NONE', *, *, #6702, .F. ) ;
#11685=CARTESIAN_POINT ( 'NONE',  ( 123.4696136271390685, -1093.703085459772637, 28.11170275877346114 ) ) ;
#11689=ORIENTED_EDGE ( 'NONE', *, *, #1195, .T. ) ;
#11707=DIRECTION ( 'NONE',  ( -1.110223024625157172E-14, 0.000000000000000000, -1.000000000000000000 ) ) ;
#11725=DIRECTION ( 'NONE',  ( 0.000000000000000000, -1.000000000000000000, 0.000000000000000000 ) ) ;
#11730=DIRECTION ( 'NONE',  ( -0.000000000000000000, -0.000000000000000000, -1.000000000000000000 ) ) ;
#11737=ORIENTED_EDGE ( 'NONE', *, *, #3708, .F. ) ;
#11745=CARTESIAN_POINT ( 'NONE',  ( -127.2684398464544415, 88.47467185906430132, 32.24990070396069086 ) ) ;
#11748=EDGE_LOOP ( 'NONE', ( #22934, #3500 ) ) ;
#11751=ORIENTED_EDGE ( 'NONE', *, *, #16705, .T. ) ;
#11753=CARTESIAN_POINT ( 'NONE',  ( 153.5653415408403646, -1122.352966361445169, 32.50000000000675726 ) ) ;
#11756=ADVANCED_FACE ( 'NONE', ( #18324 ), #18216, .F. ) ;
#11757=ADVANCED_FACE ( 'NONE', ( #23408 ), #23542, .F. ) ;
#11771=ORIENTED_EDGE ( 'NONE', *, *, #6020, .T. ) ;
#11773=CONICAL_SURFACE ( 'NONE', #6773, 2.055000000000001492, 0.7853981633974633780 ) ;
#11781=AXIS2_PLACEMENT_3D ( 'NONE', #6086, #7422, #2093 ) ;
#11783=DIRECTION ( 'NONE',  ( 0.000000000000000000, 0.000000000000000000, -1.000000000000000000 ) ) ;
#11790=VERTEX_POINT ( 'NONE', #23646 ) ;
#11798=VERTEX_POINT ( 'NONE', #1560 ) ;
#11811=ORIENTED_EDGE ( 'NONE', *, *, #19160, .T. ) ;
#11820=AXIS2_PLACEMENT_3D ( 'NONE', #18680, #8089, #20505 ) ;
#11825=EDGE_LOOP ( 'NONE', ( #23170, #1441 ) ) ;
#11828=DIRECTION ( 'NONE',  ( -1.000000000000000000, 1.408839003528726857E-14, 6.982962677686266711E-15 ) ) ;
#11839=CARTESIAN_POINT ( 'NONE',  ( 131.7935180829127830, 81.58110848117821945, 31.53271418707680240 ) ) ;
#11840=DIRECTION ( 'NONE',  ( -6.753181414994864868E-15, 6.753181414994864868E-15, -1.000000000000000000 ) ) ;
#11845=CARTESIAN_POINT ( 'NONE',  ( 155.0000000000000568, -1000.000000000000000, -90.00000000000000000 ) ) ;
#11846=DIRECTION ( 'NONE',  ( -1.350636282998972974E-14, 0.000000000000000000, -1.000000000000000000 ) ) ;
#11848=FACE_OUTER_BOUND ( 'NONE', #9816, .T. ) ;
#11851=PLANE ( 'NONE',  #5765 ) ;
#11852=DIRECTION ( 'NONE',  ( 1.000000000000000000, -1.408839003528726857E-14, -6.982962677686266711E-15 ) ) ;
#11853=FACE_OUTER_BOUND ( 'NONE', #4156, .T. ) ;
#11858=AXIS2_PLACEMENT_3D ( 'NONE', #9251, #16615, #14692 ) ;
#11884=VECTOR ( 'NONE', #16920, 1000.000000000000000 ) ;
#11891=EDGE_CURVE ( 'NONE', #17932, #21974, #16652, .T. ) ;
#11893=EDGE_LOOP ( 'NONE', ( #1086, #21393, #5454, #10224 ) ) ;
#11902=DIRECTION ( 'NONE',  ( 5.551115123125785858E-15, 0.000000000000000000, -1.000000000000000000 ) ) ;
#11906=VECTOR ( 'NONE', #5461, 1000.000000000000000 ) ;
#11915=CARTESIAN_POINT ( 'NONE',  ( 131.7919310846384633, 81.58367163796934562, -31.52881987646414430 ) ) ;
#11917=B_SPLINE_CURVE_WITH_KNOTS ( 'NONE', 3,
 ( #23372, #14001, #6606, #4430, #21328, #1026, #14112, #12315, #11839, #2952, #19145, #4784, #23136, #6473, #2607, #19622, #10004, #4544, #15910, #3090, #15790, #19380, #13885, #19502, #2840, #2741, #17369, #10491 ),
 .UNSPECIFIED., .F., .F.,
 ( 4, 2, 2, 2, 2, 2, 2, 2, 2, 2, 2, 2, 2, 4 ),
 ( 0.007862850516742146689, 0.008354729399060715003, 0.008846608281379283317, 0.009830366046016426884, 0.01032224492833498306, 0.01081412381065353923, 0.01130600269297209540, 0.01179788157529065157, 0.01278163933992775350, 0.01327351822224631314, 0.01376539710456487625, 0.01425727598688343763, 0.01474915486920199900, 0.01573291263383916339 ),
 .UNSPECIFIED. ) ;
#11920=EDGE_CURVE ( 'NONE', #12317, #6379, #4002, .T. ) ;
#11925=EDGE_CURVE ( 'NONE', #784, #10443, #23145, .T. ) ;
#11928=CARTESIAN_POINT ( 'NONE',  ( 124.4701338314437891, -1092.369831568442805, 27.50000000000646239 ) ) ;
#11931=CARTESIAN_POINT ( 'NONE',  ( -155.0000000000000284, -1000.000000000000000, -90.00000000000000000 ) ) ;
#11932=EDGE_LOOP ( 'NONE', ( #17176, #1976, #10041, #15121 ) ) ;
#11941=AXIS2_PLACEMENT_3D ( 'NONE', #10674, #1457, #21750 ) ;
#11957=CARTESIAN_POINT ( 'NONE',  ( 155.0000000000000284, 2.775557561562891351E-16, -90.00000000000000000 ) ) ;
#11970=CARTESIAN_POINT ( 'NONE',  ( 145.0000000000000568, -1000.000000000000000, -90.00000000000000000 ) ) ;
#11972=EDGE_CURVE ( 'NONE', #18892, #16653, #6613, .T. ) ;
#11973=AXIS2_PLACEMENT_3D ( 'NONE', #5039, #21571, #17581 ) ;
#11979=LINE ( 'NONE', #927, #18095 ) ;
#11985=FACE_OUTER_BOUND ( 'NONE', #5887, .T. ) ;
#11991=CIRCLE ( 'NONE', #14287, 2.499999999999998668 ) ;
#11993=EDGE_LOOP ( 'NONE', ( #10694, #16184 ) ) ;
#12004=EDGE_CURVE ( 'NONE', #9978, #7326, #14833, .T. ) ;
#12010=CIRCLE ( 'NONE', #1546, 2.055000000000001492 ) ;
#12021=AXIS2_PLACEMENT_3D ( 'NONE', #7751, #12695, #208 ) ;
#12029=ORIENTED_EDGE ( 'NONE', *, *, #2841, .F. ) ;
#12039=LINE ( 'NONE', #9949, #10175 ) ;
#12045=EDGE_CURVE ( 'NONE', #907, #12356, #19752, .T. ) ;
#12076=EDGE_CURVE ( 'NONE', #11790, #12773, #14240, .T. ) ;
#12081=FACE_OUTER_BOUND ( 'NONE', #17807, .T. ) ;
#12086=CARTESIAN_POINT ( 'NONE',  ( 126.3653543294811499, 77.28387428943223370, 32.05500000000641592 ) ) ;
#12110=DIRECTION ( 'NONE',  ( 1.000000000000000000, -1.408839003528726857E-14, -6.982962677686266711E-15 ) ) ;
#12112=CARTESIAN_POINT ( 'NONE',  ( -135.6313030678085170, -1075.027834699370487, -27.51562286569267002 ) ) ;
#12118=CARTESIAN_POINT ( 'NONE',  ( 133.0106877214038832, 79.58129789419575673, -27.51610016701188499 ) ) ;
#12121=DIRECTION ( 'NONE',  ( 1.000000000000000000, 0.000000000000000000, -0.000000000000000000 ) ) ;
#12139=DIRECTION ( 'NONE',  ( -1.000000000000000000, 1.408839003528726857E-14, 6.982962677686266711E-15 ) ) ;
#12140=VERTEX_POINT ( 'NONE', #14703 ) ;
#12151=CONICAL_SURFACE ( 'NONE', #1688, 2.055000000000001492, 0.7853981633974633780 ) ;
#12159=DIRECTION ( 'NONE',  ( 1.000000000000000000, 0.000000000000000000, -0.000000000000000000 ) ) ;
#12162=EDGE_CURVE ( 'NONE', #17788, #8566, #13029, .T. ) ;
#12166=EDGE_CURVE ( 'NONE', #3521, #16653, #23302, .T. ) ;
#12179=CARTESIAN_POINT ( 'NONE',  ( -127.9021285790841205, 87.55595642181887683, 27.50000000000646239 ) ) ;
#12189=DIRECTION ( 'NONE',  ( -0.7071067811865416886, 9.961996129952529179E-15, -0.7071067811865532349 ) ) ;
#12190=FACE_OUTER_BOUND ( 'NONE', #17387, .T. ) ;
#12191=CYLINDRICAL_SURFACE ( 'NONE', #7125, 2.500000000000002220 ) ;
#12192=CIRCLE ( 'NONE', #9450, 2.499999999999998668 ) ;
#12209=CARTESIAN_POINT ( 'NONE',  ( 0.000000000000000000, -1000.000000000000000, -90.00000000000000000 ) ) ;
#12220=CYLINDRICAL_SURFACE ( 'NONE', #9279, 145.0000000000000284 ) ;
#12231=CARTESIAN_POINT ( 'NONE',  ( 155.0000000000000284, -500.0000000000000000, -32.49999999999997158 ) ) ;
#12234=CARTESIAN_POINT ( 'NONE',  ( 133.9566469371587516, 77.97836475581189575, -31.25955389945143992 ) ) ;
#12249=DIRECTION ( 'NONE',  ( -0.7071067811865320296, 9.875400524328840493E-15, 0.7071067811865631159 ) ) ;
#12252=EDGE_CURVE ( 'NONE', #19892, #15576, #7546, .T. ) ;
#12270=DIRECTION ( 'NONE',  ( 0.000000000000000000, 0.000000000000000000, -1.000000000000000000 ) ) ;
#12276=CONICAL_SURFACE ( 'NONE', #11111, 2.055000000000001492, 0.7853981633974633780 ) ;
#12286=ORIENTED_EDGE ( 'NONE', *, *, #1028, .T. ) ;
#12296=PLANE ( 'NONE',  #371 ) ;
#12303=CARTESIAN_POINT ( 'NONE',  ( -146.0000000000000853, -494.4690652294807478, 30.00000000000641620 ) ) ;
#12310=AXIS2_PLACEMENT_3D ( 'NONE', #3520, #21519, #1704 ) ;
#12314=DIRECTION ( 'NONE',  ( -1.110223024625155594E-14, 0.000000000000000000, -1.000000000000000000 ) ) ;
#12315=CARTESIAN_POINT ( 'NONE',  ( 131.8501689178085030, 81.48954978394043280, 31.66065886938989493 ) ) ;
#12316=DIRECTION ( 'NONE',  ( 1.000000000000000000, -0.000000000000000000, 6.982962677686266711E-15 ) ) ;
#12317=VERTEX_POINT ( 'NONE', #17215 ) ;
#12318=CARTESIAN_POINT ( 'NONE',  ( -129.2206655591605511, -1072.408698320350595, 27.94500000000640227 ) ) ;
#12319=EDGE_LOOP ( 'NONE', ( #14530, #11611, #3502, #22616 ) ) ;
#12329=CYLINDRICAL_SURFACE ( 'NONE', #1815, 2.500000000000002220 ) ;
#12330=DIRECTION ( 'NONE',  ( 0.9289202219288174023, 0.3702799228849934510, 6.982962677686266711E-15 ) ) ;
#12333=CARTESIAN_POINT ( 'NONE',  ( 155.0000000000000568, -801.0618695410399823, 27.50000000000647660 ) ) ;
#12340=CARTESIAN_POINT ( 'NONE',  ( 119.6158142514525622, -1087.367367941136990, -29.99999999999356604 ) ) ;
#12348=VECTOR ( 'NONE', #19604, 1000.000000000000000 ) ;
#12355=DIRECTION ( 'NONE',  ( -1.000000000000000000, 1.408839003528726857E-14, 6.982962677686266711E-15 ) ) ;
#12356=VERTEX_POINT ( 'NONE', #8992 ) ;
#12364=EDGE_CURVE ( 'NONE', #12140, #9588, #14549, .T. ) ;
#12379=ORIENTED_EDGE ( 'NONE', *, *, #21478, .T. ) ;
#12393=DIRECTION ( 'NONE',  ( -1.000000000000000000, 1.408839003528726857E-14, 6.982962677686266711E-15 ) ) ;
#12397=DIRECTION ( 'NONE',  ( 1.000000000000000000, -0.000000000000000000, 6.982962677686266711E-15 ) ) ;
#12399=DIRECTION ( 'NONE',  ( -1.110223024625155594E-14, 0.000000000000000000, -1.000000000000000000 ) ) ;
#12404=CIRCLE ( 'NONE', #18513, 2.499999999999998668 ) ;
#12405=EDGE_CURVE ( 'NONE', #9588, #6149, #1258, .T. ) ;
#12409=CARTESIAN_POINT ( 'NONE',  ( -158.1195828810603246, 116.4077317428679947, 30.00000000000675726 ) ) ;
#12417=FACE_OUTER_BOUND ( 'NONE', #8797, .T. ) ;
#12422=CARTESIAN_POINT ( 'NONE',  ( -128.6132171834563280, 86.50814704276191947, -32.17188107257626228 ) ) ;
#12438=EDGE_LOOP ( 'NONE', ( #18435, #15930, #5352, #1899 ) ) ;
#12452=DIRECTION ( 'NONE',  ( -0.7071067811865320296, 9.875400524328840493E-15, 0.7071067811865631159 ) ) ;
#12457=DIRECTION ( 'NONE',  ( -1.110223024625155594E-14, 0.000000000000000000, -1.000000000000000000 ) ) ;
#12458=DIRECTION ( 'NONE',  ( -1.000000000000000000, -2.775557561562891351E-17, 0.000000000000000000 ) ) ;
#12459=FACE_OUTER_BOUND ( 'NONE', #4313, .T. ) ;
#12467=ORIENTED_EDGE ( 'NONE', *, *, #706, .T. ) ;
#12468=FACE_OUTER_BOUND ( 'NONE', #1690, .T. ) ;
#12470=ADVANCED_FACE ( 'NONE', ( #11304 ), #11185, .F. ) ;
#12473=EDGE_CURVE ( 'NONE', #4047, #13152, #1052, .T. ) ;
#12475=EDGE_LOOP ( 'NONE', ( #7846, #4973, #8912, #16644 ) ) ;
#12481=DIRECTION ( 'NONE',  ( 0.000000000000000000, 0.000000000000000000, -1.000000000000000000 ) ) ;
#12486=CARTESIAN_POINT ( 'NONE',  ( 133.8639378433822742, 78.13740870752386058, -28.46977261728505226 ) ) ;
#12490=CARTESIAN_POINT ( 'NONE',  ( 126.3653543294818178, 77.28387428943173632, -29.99999999999356604 ) ) ;
#12491=DIRECTION ( 'NONE',  ( 1.000000000000000000, -0.000000000000000000, 6.982962677686266711E-15 ) ) ;
#12506=DIRECTION ( 'NONE',  ( 0.000000000000000000, 5.551115123125777969E-15, -1.000000000000000000 ) ) ;
#12507=CONICAL_SURFACE ( 'NONE', #17874, 2.055000000000001492, 0.7853981633974633780 ) ;
#12519=ORIENTED_EDGE ( 'NONE', *, *, #6175, .F. ) ;
#12528=CARTESIAN_POINT ( 'NONE',  ( 153.5653415408401941, -1122.352966361446079, -32.49999999999322853 ) ) ;
#12532=CARTESIAN_POINT ( 'NONE',  ( 133.0100681275899035, 79.58233248384615877, 27.51597717546057353 ) ) ;
#12537=DIRECTION ( 'NONE',  ( -0.7071067811865416886, 9.961996129952529179E-15, -0.7071067811865532349 ) ) ;
#12538=CARTESIAN_POINT ( 'NONE',  ( 146.4449999999997658, -801.0618695410399823, 32.50000000000641620 ) ) ;
#12548=EDGE_CURVE ( 'NONE', #6763, #6579, #12039, .T. ) ;
#12566=DIRECTION ( 'NONE',  ( -2.775557561562891351E-17, 1.000000000000000000, 0.000000000000000000 ) ) ;
#12568=DIRECTION ( 'NONE',  ( 1.000000000000000000, -0.000000000000000000, 6.982962677686266711E-15 ) ) ;
#12573=AXIS2_PLACEMENT_3D ( 'NONE', #22503, #13379, #10208 ) ;
#12582=ORIENTED_EDGE ( 'NONE', *, *, #6020, .F. ) ;
#12594=CARTESIAN_POINT ( 'NONE',  ( 134.0610795706244858, 77.79865694966356671, -29.19154146838981134 ) ) ;
#12599=CARTESIAN_POINT ( 'NONE',  ( -126.4561707720353354, 89.63167338449116528, -30.32927184981475222 ) ) ;
#12623=DIRECTION ( 'NONE',  ( 6.580500949201931673E-15, 2.336402151923303105E-15, 1.000000000000000000 ) ) ;
#12638=DIRECTION ( 'NONE',  ( 0.7232617928448825673, -0.6905739489807055653, -6.982962677686266711E-15 ) ) ;
#12644=CARTESIAN_POINT ( 'NONE',  ( 124.6683470056599106, -1092.102735484116010, 27.50000000000645173 ) ) ;
#12646=CONICAL_SURFACE ( 'NONE', #2174, 2.055000000000001492, 0.7853981633974633780 ) ;
#12653=DIRECTION ( 'NONE',  ( 1.000000000000000000, 0.000000000000000000, -0.000000000000000000 ) ) ;
#12667=ORIENTED_EDGE ( 'NONE', *, *, #6926, .F. ) ;
#12675=CONICAL_SURFACE ( 'NONE', #7208, 2.055000000000001492, 0.7853981633974633780 ) ;
#12678=DIRECTION ( 'NONE',  ( -0.000000000000000000, -0.000000000000000000, -1.000000000000000000 ) ) ;
#12690=ORIENTED_EDGE ( 'NONE', *, *, #21075, .T. ) ;
#12695=DIRECTION ( 'NONE',  ( -1.000000000000000000, 1.408839003528726857E-14, 6.982962677686266711E-15 ) ) ;
#12700=DIRECTION ( 'NONE',  ( 5.551115123125785858E-15, 0.000000000000000000, -1.000000000000000000 ) ) ;
#12701=ORIENTED_EDGE ( 'NONE', *, *, #11541, .T. ) ;
#12703=VECTOR ( 'NONE', #19867, 1000.000000000000114 ) ;
#12708=CARTESIAN_POINT ( 'NONE',  ( 119.9257125005557327, -1087.686723660050802, -32.49999999999356959 ) ) ;
#12714=CARTESIAN_POINT ( 'NONE',  ( -127.4426065742854064, 88.22361005463105244, -27.62591505085368482 ) ) ;
#12735=CIRCLE ( 'NONE', #18838, 2.499999999999998668 ) ;
#12739=AXIS2_PLACEMENT_3D ( 'NONE', #20873, #19039, #2504 ) ;
#12742=VECTOR ( 'NONE', #20974, 1000.000000000000000 ) ;
#12759=DIRECTION ( 'NONE',  ( -6.753181414994864868E-15, 6.753181414994864868E-15, -1.000000000000000000 ) ) ;
#12761=CONICAL_SURFACE ( 'NONE', #17734, 2.055000000000001492, 0.7853981633974633780 ) ;
#12764=EDGE_CURVE ( 'NONE', #14056, #18892, #20195, .T. ) ;
#12773=VERTEX_POINT ( 'NONE', #6976 ) ;
#12774=VERTEX_POINT ( 'NONE', #18194 ) ;
#12776=CARTESIAN_POINT ( 'NONE',  ( 125.3835310783086356, -1091.126227143374535, 28.00959664470840238 ) ) ;
#12779=EDGE_CURVE ( 'NONE', #16229, #7198, #1299, .T. ) ;
#12780=CARTESIAN_POINT ( 'NONE',  ( -129.3177328886530120, 85.45129583908924076, 30.16873261443288001 ) ) ;
#12783=CARTESIAN_POINT ( 'NONE',  ( 133.8639378433819047, 78.13740870752447165, 31.53022738271491576 ) ) ;
#12785=CONICAL_SURFACE ( 'NONE', #13178, 2.055000000000001492, 0.7853981633974633780 ) ;
#12788=DIRECTION ( 'NONE',  ( -1.000000000000000000, 1.408839003528726857E-14, 6.982962677686266711E-15 ) ) ;
#12799=CIRCLE ( 'NONE', #15851, 2.499999999999998668 ) ;
#12803=CARTESIAN_POINT ( 'NONE',  ( 146.4449999999997942, -209.9999999999996874, 27.50000000000642331 ) ) ;
#12806=EDGE_LOOP ( 'NONE', ( #8373, #17453, #20650, #5117 ) ) ;
#12812=CARTESIAN_POINT ( 'NONE',  ( 123.7129353098586932, -1093.381627813014120, -27.82770220384456650 ) ) ;
#12823=CARTESIAN_POINT ( 'NONE',  ( 119.6158142514527469, -1087.367367941136308, 27.94500000000641293 ) ) ;
#12824=CARTESIAN_POINT ( 'NONE',  ( -194.7500000000000284, -784.4690652294799520, 30.00000000000675726 ) ) ;
#12832=CARTESIAN_POINT ( 'NONE',  ( -194.7500000000004547, -784.4690652294792699, -27.49999999999322498 ) ) ;
#12833=CARTESIAN_POINT ( 'NONE',  ( -136.5243927815876361, -1073.390114808524004, 31.99235058689517430 ) ) ;
#12837=DIRECTION ( 'NONE',  ( -1.000000000000000000, 1.408839003528726857E-14, 6.982962677686266711E-15 ) ) ;
#12844=LINE ( 'NONE', #11129, #16854 ) ;
#12860=CYLINDRICAL_SURFACE ( 'NONE', #314, 2.500000000000002220 ) ;
#12861=CARTESIAN_POINT ( 'NONE',  ( 124.8644691973859295, -1091.836575763270957, -32.43450926607476248 ) ) ;
#12866=CIRCLE ( 'NONE', #21683, 2.055000000000001492 ) ;
#12874=CARTESIAN_POINT ( 'NONE',  ( 119.6158142514525764, -1087.367367941136990, -32.05499999999357641 ) ) ;
#12877=FACE_OUTER_BOUND ( 'NONE', #11932, .T. ) ;
#12882=CARTESIAN_POINT ( 'NONE',  ( 125.9653219304451000, -1090.320195256218767, 29.67150201188739089 ) ) ;
#12885=CARTESIAN_POINT ( 'NONE',  ( 132.8404720734530144, 79.86494211668951948, 32.50000000000646594 ) ) ;
#12891=ADVANCED_FACE ( 'NONE', ( #12459 ), #12151, .F. ) ;
#12896=DIRECTION ( 'NONE',  ( -0.9289202219288174023, -0.3702799228849933955, -6.982962677686267499E-15 ) ) ;
#12898=EDGE_LOOP ( 'NONE', ( #19320, #1712 ) ) ;
#12909=DIRECTION ( 'NONE',  ( 1.000000000000000000, 0.000000000000000000, 0.000000000000000000 ) ) ;
#12913=CARTESIAN_POINT ( 'NONE',  ( 123.5484583266983094, -1093.599130927305623, -31.99339931332756493 ) ) ;
#12916=CARTESIAN_POINT ( 'NONE',  ( -122.8605704798722940, 82.74225173005859801, 32.05500000000641592 ) ) ;
#12918=DIRECTION ( 'NONE',  ( -0.9423651898111409242, -0.3345860861306287903, 6.982962677686267499E-15 ) ) ;
#12919=ORIENTED_EDGE ( 'NONE', *, *, #8132, .F. ) ;
#12922=DIRECTION ( 'NONE',  ( 1.000000000000000000, -0.000000000000000000, 6.982962677686266711E-15 ) ) ;
#12930=ADVANCED_FACE ( 'NONE', ( #22274 ), #7798, .F. ) ;
#12942=DIRECTION ( 'NONE',  ( 0.000000000000000000, 0.000000000000000000, -1.000000000000000000 ) ) ;
#12946=AXIS2_PLACEMENT_3D ( 'NONE', #16625, #4157, #20699 ) ;
#12951=CARTESIAN_POINT ( 'NONE',  ( -158.1195828810603246, 116.4077317428679805, 32.50000000000675726 ) ) ;
#12953=VERTEX_POINT ( 'NONE', #20580 ) ;
#12959=ADVANCED_FACE ( 'NONE', ( #83 ), #3919, .F. ) ;
#12960=CARTESIAN_POINT ( 'NONE',  ( 146.0000000000002274, -801.0618695410406644, -29.99999999999356604 ) ) ;
#12968=LINE ( 'NONE', #12528, #20029 ) ;
#12970=CIRCLE ( 'NONE', #11820, 2.055000000000001492 ) ;
#12973=CARTESIAN_POINT ( 'NONE',  ( 125.9653219304447447, -1090.320195256219449, -30.32849798811274411 ) ) ;
#12979=AXIS2_PLACEMENT_3D ( 'NONE', #22204, #2403, #20396 ) ;
#12984=CARTESIAN_POINT ( 'NONE',  ( -135.9481979339309135, -1074.452087582500099, -32.48402282453943002 ) ) ;
#12994=DIRECTION ( 'NONE',  ( -1.000000000000000000, 0.000000000000000000, -6.982962677686266711E-15 ) ) ;
#12995=CARTESIAN_POINT ( 'NONE',  ( -129.6400180686265173, -1072.557589128678728, 30.00000000000641975 ) ) ;
#13022=VECTOR ( 'NONE', #10477, 1000.000000000000000 ) ;
#13025=ADVANCED_FACE ( 'NONE', ( #20224 ), #7676, .F. ) ;
#13026=VERTEX_POINT ( 'NONE', #22154 ) ;
#13029=LINE ( 'NONE', #20331, #15997 ) ;
#13033=CARTESIAN_POINT ( 'NONE',  ( 122.9957307409590186, -1094.324181863848480, -29.34813586885355363 ) ) ;
#13036=DIRECTION ( 'NONE',  ( 1.000000000000000000, -0.000000000000000000, -0.000000000000000000 ) ) ;
#13043=FACE_OUTER_BOUND ( 'NONE', #18186, .T. ) ;
#13046=ORIENTED_EDGE ( 'NONE', *, *, #871, .T. ) ;
#13050=ORIENTED_EDGE ( 'NONE', *, *, #14215, .T. ) ;
#13055=ORIENTED_EDGE ( 'NONE', *, *, #22522, .T. ) ;
#13096=CARTESIAN_POINT ( 'NONE',  ( 124.4701338314433201, -1092.369831568443260, -32.49999999999351985 ) ) ;
#13098=EDGE_CURVE ( 'NONE', #14948, #17788, #2490, .T. ) ;
#13101=CARTESIAN_POINT ( 'NONE',  ( 119.6158142514527469, -1087.367367941136308, 27.94500000000641649 ) ) ;
#13106=CARTESIAN_POINT ( 'NONE',  ( -136.5854636148305019, -1073.276359373527612, -31.88829724122658860 ) ) ;
#13113=VERTEX_POINT ( 'NONE', #4409 ) ;
#13124=CARTESIAN_POINT ( 'NONE',  ( 125.8126197883822641, -1090.532805371500217, 31.11671059283543528 ) ) ;
#13126=CARTESIAN_POINT ( 'NONE',  ( -129.1735827702802055, 85.66907061909537902, 31.11671059283535712 ) ) ;
#13130=CIRCLE ( 'NONE', #2668, 2.499999999999998668 ) ;
#13132=CARTESIAN_POINT ( 'NONE',  ( 155.0000000000000284, -500.0000000000000000, -29.99999999999997158 ) ) ;
#13139=CONICAL_SURFACE ( 'NONE', #4592, 2.055000000000001492, 0.7853981633974633780 ) ;
#13143=CARTESIAN_POINT ( 'NONE',  ( 132.1831532210149476, 80.94878845338332951, -27.81095155082709525 ) ) ;
#13152=VERTEX_POINT ( 'NONE', #12179 ) ;
#13159=DIRECTION ( 'NONE',  ( -0.9423651898111409242, -0.3345860861306287903, 6.982962677686267499E-15 ) ) ;
#13162=CARTESIAN_POINT ( 'NONE',  ( 123.1514321905979443, -1094.120844545942873, -31.25955389945132268 ) ) ;
#13178=AXIS2_PLACEMENT_3D ( 'NONE', #11232, #2115, #677 ) ;
#13190=DIRECTION ( 'NONE',  ( 0.000000000000000000, 0.000000000000000000, 1.000000000000000000 ) ) ;
#13201=CARTESIAN_POINT ( 'NONE',  ( 146.0000000000002274, -210.0000000000003411, -29.99999999999356604 ) ) ;
#13213=DIRECTION ( 'NONE',  ( 0.000000000000000000, 0.000000000000000000, -1.000000000000000000 ) ) ;
#13214=FACE_OUTER_BOUND ( 'NONE', #15092, .T. ) ;
#13216=CARTESIAN_POINT ( 'NONE',  ( -129.0269476471444534, 85.88978664864571044, -28.46728581292316207 ) ) ;
#13230=CARTESIAN_POINT ( 'NONE',  ( -135.1739945062388415, -1075.849084086416042, 32.18904844917291541 ) ) ;
#13237=DIRECTION ( 'NONE',  ( 1.000000000000000000, -0.000000000000000000, 6.982962677686266711E-15 ) ) ;
#13240=ORIENTED_EDGE ( 'NONE', *, *, #19348, .F. ) ;
#13242=CARTESIAN_POINT ( 'NONE',  ( 119.9257125005558606, -1087.686723660049893, 30.00000000000641975 ) ) ;
#13244=CARTESIAN_POINT ( 'NONE',  ( -129.1300454301538707, 85.73470730629014724, 31.26048023074367421 ) ) ;
#13255=DIRECTION ( 'NONE',  ( 1.000000000000000000, -0.000000000000000000, 6.982962677686266711E-15 ) ) ;
#13258=AXIS2_PLACEMENT_3D ( 'NONE', #22073, #9059, #20257 ) ;
#13260=CARTESIAN_POINT ( 'NONE',  ( 124.0809974055277678, -1092.892044598689608, 27.57867027829822959 ) ) ;
#13289=ORIENTED_EDGE ( 'NONE', *, *, #18314, .F. ) ;
#13306=AXIS2_PLACEMENT_3D ( 'NONE', #15303, #18539, #16739 ) ;
#13318=EDGE_CURVE ( 'NONE', #9978, #16229, #23596, .T. ) ;
#13319=CYLINDRICAL_SURFACE ( 'NONE', #23664, 2.500000000000002220 ) ;
#13322=CARTESIAN_POINT ( 'NONE',  ( 126.7787238282401461, 77.44864885511553609, -29.99999999999356248 ) ) ;
#13332=LINE ( 'NONE', #13101, #16113 ) ;
#13344=FACE_OUTER_BOUND ( 'NONE', #825, .T. ) ;
#13345=ORIENTED_EDGE ( 'NONE', *, *, #22168, .F. ) ;
#13346=CARTESIAN_POINT ( 'NONE',  ( 145.9999999999998010, -801.0618695410399823, 30.00000000000641620 ) ) ;
#13363=ADVANCED_FACE ( 'NONE', ( #166 ), #19043, .F. ) ;
#13377=CARTESIAN_POINT ( 'NONE',  ( 122.9870427404262045, -1094.335589877584425, 29.33965772977896691 ) ) ;
#13379=DIRECTION ( 'NONE',  ( 1.000000000000000000, -0.000000000000000000, 6.982962677686266711E-15 ) ) ;
#13381=FACE_BOUND ( 'NONE', #3876, .T. ) ;
#13387=ORIENTED_EDGE ( 'NONE', *, *, #21677, .T. ) ;
#13416=DIRECTION ( 'NONE',  ( 1.000000000000000000, -0.000000000000000000, 6.982962677686266711E-15 ) ) ;
#13426=FACE_OUTER_BOUND ( 'NONE', #3682, .T. ) ;
#13441=ORIENTED_EDGE ( 'NONE', *, *, #6670, .F. ) ;
#13449=B_SPLINE_CURVE_WITH_KNOTS ( 'NONE', 3,
 ( #2425, #11167, #14891, #6050, #13466, #13230, #7621, #18962, #9814, #11521, #20537, #1953, #9341, #150, #22225, #5696, #11401, #3882, #18601, #18717, #2177, #17055, #9566, #16931, #5936, #17169, #401, #7760 ),
 .UNSPECIFIED., .F., .F.,
 ( 4, 2, 2, 2, 2, 2, 2, 2, 2, 2, 2, 2, 2, 4 ),
 ( 0.007862850516741886481, 0.008354729399060628267, 0.008846608281379370053, 0.009830366046016853626, 0.01032224492833538204, 0.01081412381065390872, 0.01130600269297243540, 0.01179788157529096382, 0.01278163933992802759, 0.01327351822224656294, 0.01376539710456510177, 0.01425727598688363712, 0.01474915486920217247, 0.01573291263383924665 ),
 .UNSPECIFIED. ) ;
#13454=EDGE_CURVE ( 'NONE', #10574, #12356, #2079, .T. ) ;
#13462=CARTESIAN_POINT ( 'NONE',  ( -136.1788113199118584, -1074.029417785592386, -32.37389708099358643 ) ) ;
#13466=CARTESIAN_POINT ( 'NONE',  ( -135.3962747006860354, -1075.451122483741756, 32.37380477188061434 ) ) ;
#13508=CARTESIAN_POINT ( 'NONE',  ( 123.8018707182401101, -1093.263712923000639, 32.24990070396069086 ) ) ;
#13512=AXIS2_PLACEMENT_3D ( 'NONE', #20949, #5860, #5746 ) ;
#13543=AXIS2_PLACEMENT_3D ( 'NONE', #8800, #12922, #8930 ) ;
#13546=CARTESIAN_POINT ( 'NONE',  ( 126.3653543294811499, 77.28387428943223370, 27.94500000000641649 ) ) ;
#13563=VECTOR ( 'NONE', #5824, 1000.000000000000114 ) ;
#13573=CARTESIAN_POINT ( 'NONE',  ( -127.1852154257921086, 88.59424271557165298, 27.82653936295257324 ) ) ;
#13575=ORIENTED_EDGE ( 'NONE', *, *, #5297, .F. ) ;
#13600=EDGE_CURVE ( 'NONE', #21974, #5229, #21554, .T. ) ;
#13604=ORIENTED_EDGE ( 'NONE', *, *, #12076, .T. ) ;
#13612=( NAMED_UNIT ( * ) SI_UNIT ( $, .STERADIAN. ) SOLID_ANGLE_UNIT ( ) );
#13620=ORIENTED_EDGE ( 'NONE', *, *, #1857, .F. ) ;
#13624=CARTESIAN_POINT ( 'NONE',  ( 122.9459112154328579, -1094.389103796012705, 30.16266818053248500 ) ) ;
#13626=ORIENTED_EDGE ( 'NONE', *, *, #22720, .T. ) ;
#13631=DIRECTION ( 'NONE',  ( -0.9423651898111408132, -0.3345860861306287348, 6.982962677686266711E-15 ) ) ;
#13643=PLANE ( 'NONE',  #11596 ) ;
#13655=FACE_OUTER_BOUND ( 'NONE', #9879, .T. ) ;
#13656=ORIENTED_EDGE ( 'NONE', *, *, #11541, .F. ) ;
#13669=DIRECTION ( 'NONE',  ( 6.982962677686266711E-15, -9.837870180509810443E-29, 1.000000000000000000 ) ) ;
#13682=CARTESIAN_POINT ( 'NONE',  ( -127.1840658299263112, 88.59589253999637037, 32.17229779615544771 ) ) ;
#13701=EDGE_CURVE ( 'NONE', #10033, #21432, #8840, .T. ) ;
#13739=EDGE_LOOP ( 'NONE', ( #23188, #6836, #18875, #717 ) ) ;
#13741=VERTEX_POINT ( 'NONE', #17646 ) ;
#13751=FACE_OUTER_BOUND ( 'NONE', #15882, .T. ) ;
#13758=ORIENTED_EDGE ( 'NONE', *, *, #14467, .F. ) ;
#13761=VECTOR ( 'NONE', #5799, 1000.000000000000000 ) ;
#13763=DIRECTION ( 'NONE',  ( 1.000000000000000000, -0.000000000000000000, 6.982962677686266711E-15 ) ) ;
#13764=ADVANCED_FACE ( 'NONE', ( #18016 ), #10798, .F. ) ;
#13766=DIRECTION ( 'NONE',  ( -2.775557561562891351E-17, 1.000000000000000000, 0.000000000000000000 ) ) ;
#13768=AXIS2_PLACEMENT_3D ( 'NONE', #18532, #439, #1986 ) ;
#13797=ORIENTED_EDGE ( 'NONE', *, *, #16362, .F. ) ;
#13803=ORIENTED_EDGE ( 'NONE', *, *, #3122, .F. ) ;
#13824=DIRECTION ( 'NONE',  ( 6.753181414994864868E-15, 0.000000000000000000, -1.000000000000000000 ) ) ;
#13833=CIRCLE ( 'NONE', #3367, 2.500000000000002220 ) ;
#13840=VERTEX_POINT ( 'NONE', #11389 ) ;
#13848=CIRCLE ( 'NONE', #11941, 2.500000000000002220 ) ;
#13855=CARTESIAN_POINT ( 'NONE',  ( -146.4450000000000784, -784.4690652294805204, 30.00000000000641975 ) ) ;
#13859=DIRECTION ( 'NONE',  ( -1.110223024625157172E-14, 0.000000000000000000, -1.000000000000000000 ) ) ;
#13872=CONICAL_SURFACE ( 'NONE', #10776, 2.055000000000001492, 0.7853981633974633780 ) ;
#13881=DIRECTION ( 'NONE',  ( 0.000000000000000000, 5.551115123125777969E-15, -1.000000000000000000 ) ) ;
#13885=CARTESIAN_POINT ( 'NONE',  ( 132.0389103176321441, 81.18340533128269954, 28.00959664470845567 ) ) ;
#13897=CIRCLE ( 'NONE', #15404, 2.500000000000002220 ) ;
#13899=VERTEX_POINT ( 'NONE', #20524 ) ;
#13910=AXIS2_PLACEMENT_3D ( 'NONE', #16186, #23546, #7002 ) ;
#13918=AXIS2_PLACEMENT_3D ( 'NONE', #19748, #7069, #6835 ) ;
#13933=CONICAL_SURFACE ( 'NONE', #8886, 2.055000000000001492, 0.7853981633974633780 ) ;
#13937=DIRECTION ( 'NONE',  ( 1.000000000000000000, -0.000000000000000000, 6.982962677686266711E-15 ) ) ;
#13950=ORIENTED_EDGE ( 'NONE', *, *, #12779, .T. ) ;
#13978=PLANE ( 'NONE',  #2091 ) ;
#13984=CARTESIAN_POINT ( 'NONE',  ( 119.6158142514527327, -1087.367367941136308, 30.00000000000641620 ) ) ;
#13991=DIRECTION ( 'NONE',  ( -1.000000000000000000, 1.408839003528726857E-14, 6.982962677686266711E-15 ) ) ;
#14001=CARTESIAN_POINT ( 'NONE',  ( 132.7558223547125067, 80.00574117445309241, 32.50000000000647304 ) ) ;
#14005=CARTESIAN_POINT ( 'NONE',  ( -194.7500000000000284, -204.4690652294800657, 30.00000000000675726 ) ) ;
#14010=DIRECTION ( 'NONE',  ( 1.000000000000000000, 0.000000000000000000, 0.000000000000000000 ) ) ;
#14013=PLANE ( 'NONE',  #16935 ) ;
#14027=CARTESIAN_POINT ( 'NONE',  ( -126.5312127422334498, 89.52572971382257094, 30.80845853161017800 ) ) ;
#14031=AXIS2_PLACEMENT_3D ( 'NONE', #3000, #12491, #2878 ) ;
#14032=ORIENTED_EDGE ( 'NONE', *, *, #10132, .T. ) ;
#14037=CARTESIAN_POINT ( 'NONE',  ( 133.4124711242730541, 78.90586732742340814, -32.24959887471651854 ) ) ;
#14050=EDGE_LOOP ( 'NONE', ( #16097, #21714, #3344, #19685 ) ) ;
#14056=VERTEX_POINT ( 'NONE', #9924 ) ;
#14060=EDGE_CURVE ( 'NONE', #6254, #17523, #22337, .T. ) ;
#14086=ORIENTED_EDGE ( 'NONE', *, *, #23180, .T. ) ;
#14093=DIRECTION ( 'NONE',  ( -1.000000000000000000, 1.408839003528726857E-14, 6.982962677686266711E-15 ) ) ;
#14098=DIRECTION ( 'NONE',  ( -0.6964005597823108573, 0.7176533009294141507, -6.982962677686267499E-15 ) ) ;
#14112=CARTESIAN_POINT ( 'NONE',  ( 132.0350058597967404, 81.18997658688670072, 32.00444854364500458 ) ) ;
#14116=ORIENTED_EDGE ( 'NONE', *, *, #17472, .F. ) ;
#14123=FACE_OUTER_BOUND ( 'NONE', #21452, .T. ) ;
#14133=ORIENTED_EDGE ( 'NONE', *, *, #1028, .F. ) ;
#14147=ORIENTED_EDGE ( 'NONE', *, *, #15346, .F. ) ;
#14152=DIRECTION ( 'NONE',  ( -0.7232617928448825673, 0.6905739489807055653, 6.982962677686266711E-15 ) ) ;
#14162=ORIENTED_EDGE ( 'NONE', *, *, #8374, .F. ) ;
#14175=EDGE_CURVE ( 'NONE', #10443, #45, #15794, .T. ) ;
#14178=DIRECTION ( 'NONE',  ( 1.110223024625157172E-14, 0.000000000000000000, -1.000000000000000000 ) ) ;
#14185=ORIENTED_EDGE ( 'NONE', *, *, #8157, .F. ) ;
#14188=LINE ( 'NONE', #20072, #11906 ) ;
#14199=CIRCLE ( 'NONE', #16877, 2.055000000000001492 ) ;
#14202=VERTEX_POINT ( 'NONE', #22295 ) ;
#14203=CARTESIAN_POINT ( 'NONE',  ( -128.8385278530642495, 86.17219694792784423, -31.88744336596579387 ) ) ;
#14204=CARTESIAN_POINT ( 'NONE',  ( -145.0000000000000284, -1000.000000000000000, -90.00000000000000000 ) ) ;
#14207=CARTESIAN_POINT ( 'NONE',  ( 119.9257125005558891, -1087.686723660049893, 27.50000000000641975 ) ) ;
#14215=EDGE_CURVE ( 'NONE', #21432, #10033, #22718, .T. ) ;
#14223=VERTEX_POINT ( 'NONE', #2127 ) ;
#14235=EDGE_LOOP ( 'NONE', ( #4583, #22496, #22237, #11323 ) ) ;
#14240=LINE ( 'NONE', #3098, #9812 ) ;
#14247=DIRECTION ( 'NONE',  ( -1.110223024625157172E-14, 0.000000000000000000, -1.000000000000000000 ) ) ;
#14249=CYLINDRICAL_SURFACE ( 'NONE', #23091, 2.500000000000002220 ) ;
#14263=CIRCLE ( 'NONE', #12739, 2.055000000000001492 ) ;
#14268=ORIENTED_EDGE ( 'NONE', *, *, #14355, .F. ) ;
#14269=CARTESIAN_POINT ( 'NONE',  ( -134.6777706902594787, -1076.726150876685324, -28.88328940716457893 ) ) ;
#14276=CARTESIAN_POINT ( 'NONE',  ( -129.2206655591605511, -1072.408698320350595, 27.94500000000641649 ) ) ;
#14287=AXIS2_PLACEMENT_3D ( 'NONE', #13855, #21878, #3757 ) ;
#14289=ORIENTED_EDGE ( 'NONE', *, *, #18033, .F. ) ;
#14293=CARTESIAN_POINT ( 'NONE',  ( 194.7500000000002274, -210.0000000000003411, -32.49999999999322853 ) ) ;
#14296=ORIENTED_EDGE ( 'NONE', *, *, #706, .F. ) ;
#14334=CARTESIAN_POINT ( 'NONE',  ( -128.7674363984956756, 86.27842408395288487, -31.99040335529151946 ) ) ;
#14337=CARTESIAN_POINT ( 'NONE',  ( 133.4862419878492688, 78.78097527456812088, 27.82653936295257324 ) ) ;
#14340=FACE_OUTER_BOUND ( 'NONE', #15023, .T. ) ;
#14355=EDGE_CURVE ( 'NONE', #404, #14202, #361, .T. ) ;
#14362=DIRECTION ( 'NONE',  ( -0.9423651898111409242, -0.3345860861306287903, 6.982962677686267499E-15 ) ) ;
#14365=EDGE_CURVE ( 'NONE', #9157, #963, #8193, .T. ) ;
#14379=PLANE ( 'NONE',  #21122 ) ;
#14385=ORIENTED_EDGE ( 'NONE', *, *, #5363, .F. ) ;
#14391=CONICAL_SURFACE ( 'NONE', #1252, 2.055000000000001492, 0.7853981633974633780 ) ;
#14393=CARTESIAN_POINT ( 'NONE',  ( -126.9531799701276213, 88.92639545932848932, -31.88829724122659570 ) ) ;
#14396=DIRECTION ( 'NONE',  ( 0.000000000000000000, 0.000000000000000000, -1.000000000000000000 ) ) ;
#14422=VERTEX_POINT ( 'NONE', #12318 ) ;
#14425=EDGE_LOOP ( 'NONE', ( #3051, #283, #3915, #5923 ) ) ;
#14426=PLANE ( 'NONE',  #18393 ) ;
#14427=VERTEX_POINT ( 'NONE', #21447 ) ;
#14434=EDGE_CURVE ( 'NONE', #16240, #8499, #2699, .T. ) ;
#14443=CARTESIAN_POINT ( 'NONE',  ( -146.4450000000005332, -784.4690652294799520, -29.99999999999356248 ) ) ;
#14450=LINE ( 'NONE', #22134, #20808 ) ;
#14452=CARTESIAN_POINT ( 'NONE',  ( 155.0000000000000568, -801.0618695410406644, -29.99999999999350564 ) ) ;
#14457=ORIENTED_EDGE ( 'NONE', *, *, #871, .F. ) ;
#14458=CARTESIAN_POINT ( 'NONE',  ( 155.0000000000000568, -801.0618695410406644, -29.99999999999350564 ) ) ;
#14463=( NAMED_UNIT ( * ) SI_UNIT ( $, .STERADIAN. ) SOLID_ANGLE_UNIT ( ) );
#14464=DIRECTION ( 'NONE',  ( 0.000000000000000000, 0.000000000000000000, -1.000000000000000000 ) ) ;
#14467=EDGE_CURVE ( 'NONE', #4130, #14975, #9261, .T. ) ;
#14471=ORIENTED_EDGE ( 'NONE', *, *, #16202, .F. ) ;
#14476=ADVANCED_FACE ( 'NONE', ( #5143 ), #12761, .F. ) ;
#14477=ORIENTED_EDGE ( 'NONE', *, *, #1862, .T. ) ;
#14483=EDGE_LOOP ( 'NONE', ( #19837, #1014 ) ) ;
#14488=AXIS2_PLACEMENT_3D ( 'NONE', #3579, #9289, #5644 ) ;
#14497=CARTESIAN_POINT ( 'NONE',  ( -126.6052862049306924, 89.42094583968793131, -31.11320915316591851 ) ) ;
#14499=FACE_BOUND ( 'NONE', #2867, .T. ) ;
#14505=EDGE_CURVE ( 'NONE', #21432, #16240, #1168, .T. ) ;
#14522=DIRECTION ( 'NONE',  ( 0.7232617928448825673, -0.6905739489807055653, -6.982962677686266711E-15 ) ) ;
#14530=ORIENTED_EDGE ( 'NONE', *, *, #15687, .F. ) ;
#14535=ORIENTED_EDGE ( 'NONE', *, *, #2806, .F. ) ;
#14536=DIRECTION ( 'NONE',  ( 1.000000000000000000, 0.000000000000000000, -0.000000000000000000 ) ) ;
#14549=LINE ( 'NONE', #10832, #4367 ) ;
#14550=CARTESIAN_POINT ( 'NONE',  ( 133.9566469371582684, 77.97836475581249260, 28.74044610054856008 ) ) ;
#14575=CARTESIAN_POINT ( 'NONE',  ( 123.2641556675335437, -1093.973169342143592, -31.53250949154602623 ) ) ;
#14597=EDGE_CURVE ( 'NONE', #22831, #19928, #8315, .T. ) ;
#14608=CARTESIAN_POINT ( 'NONE',  ( -146.4450000000005332, -204.4690652294800657, -29.99999999999356248 ) ) ;
#14610=CARTESIAN_POINT ( 'NONE',  ( -127.9021285790837510, 87.55595642181940264, -27.49999999999351985 ) ) ;
#14611=CARTESIAN_POINT ( 'NONE',  ( 124.4701338314433201, -1092.369831568443260, -32.49999999999351985 ) ) ;
#14619=AXIS2_PLACEMENT_3D ( 'NONE', #19751, #3199, #21333 ) ;
#14644=EDGE_CURVE ( 'NONE', #6149, #4706, #19272, .T. ) ;
#14659=CIRCLE ( 'NONE', #8887, 2.500000000000002220 ) ;
#14670=CARTESIAN_POINT ( 'NONE',  ( 125.3881179880848293, -1091.120112697373088, 32.00444854364510405 ) ) ;
#14673=CARTESIAN_POINT ( 'NONE',  ( -129.2722218393576554, 85.52013646629063714, 30.65375098132849274 ) ) ;
#14674=AXIS2_PLACEMENT_3D ( 'NONE', #10296, #2893, #17520 ) ;
#14681=EDGE_CURVE ( 'NONE', #15889, #9157, #14659, .T. ) ;
#14692=DIRECTION ( 'NONE',  ( 1.350636282998972974E-14, 0.000000000000000000, -1.000000000000000000 ) ) ;
#14700=DIRECTION ( 'NONE',  ( 0.000000000000000000, 0.000000000000000000, -1.000000000000000000 ) ) ;
#14703=CARTESIAN_POINT ( 'NONE',  ( -146.0000000000005400, -784.4690652294799520, -32.05499999999356930 ) ) ;
#14705=CARTESIAN_POINT ( 'NONE',  ( 124.4701338314433485, -1092.369831568443260, -27.49999999999351985 ) ) ;
#14714=ORIENTED_EDGE ( 'NONE', *, *, #12004, .T. ) ;
#14718=DIRECTION ( 'NONE',  ( 0.6568457881071649851, 0.2618274444092050790, 0.7071067811865631159 ) ) ;
#14735=DIRECTION ( 'NONE',  ( -1.110223024625157172E-14, 0.000000000000000000, -1.000000000000000000 ) ) ;
#14737=CARTESIAN_POINT ( 'NONE',  ( -127.7150463208621716, 87.82877071840164263, -27.51610016701188499 ) ) ;
#14742=CARTESIAN_POINT ( 'NONE',  ( 155.0000000000000568, -801.0618695410406644, -32.49999999999350564 ) ) ;
#14750=ORIENTED_EDGE ( 'NONE', *, *, #14060, .T. ) ;
#14754=CARTESIAN_POINT ( 'NONE',  ( -128.3589811823731281, 86.88495287852444449, -27.62619522811937856 ) ) ;
#14761=ORIENTED_EDGE ( 'NONE', *, *, #16864, .T. ) ;
#14769=CARTESIAN_POINT ( 'NONE',  ( -136.9911991620665788, -1072.514904345033074, -30.32927184981475577 ) ) ;
#14774=DIRECTION ( 'NONE',  ( 1.110223024625155594E-14, 0.000000000000000000, -1.000000000000000000 ) ) ;
#14777=EDGE_CURVE ( 'NONE', #22609, #12140, #12010, .T. ) ;
#14787=CARTESIAN_POINT ( 'NONE',  ( 124.9522429225340545, -1091.716738251577226, 32.37380477188062144 ) ) ;
#14789=CARTESIAN_POINT ( 'NONE',  ( 171.6502151485109664, 95.33502053007563859, 30.00000000000675726 ) ) ;
#14790=CARTESIAN_POINT ( 'NONE',  ( 132.8404720734530144, 79.86494211668949106, 27.50000000000646239 ) ) ;
#14800=CARTESIAN_POINT ( 'NONE',  ( 131.5158088764654565, 82.02799531629160867, -29.83126738556711288 ) ) ;
#14805=EDGE_CURVE ( 'NONE', #15996, #14223, #16957, .T. ) ;
#14817=CARTESIAN_POINT ( 'NONE',  ( -155.0000000000000284, -784.4690652294799520, -27.49999999999350209 ) ) ;
#14821=CARTESIAN_POINT ( 'NONE',  ( 123.1512869713293554, -1094.121033843497344, -28.74099766568595982 ) ) ;
#14822=CARTESIAN_POINT ( 'NONE',  ( 145.9999999999998295, -801.0618695410399823, 27.94500000000641649 ) ) ;
#14833=CIRCLE ( 'NONE', #17511, 2.055000000000001492 ) ;
#14842=CARTESIAN_POINT ( 'NONE',  ( 0.000000000000000000, -1000.000000000000000, 90.00000000000000000 ) ) ;
#14846=DIRECTION ( 'NONE',  ( -0.7232617928448825673, 0.6905739489807055653, 6.982962677686265922E-15 ) ) ;
#14856=CARTESIAN_POINT ( 'NONE',  ( -146.0000000000000568, -494.4690652294807478, 32.05500000000641592 ) ) ;
#14865=DIRECTION ( 'NONE',  ( -1.000000000000000000, 1.408839003528726857E-14, 6.982962677686266711E-15 ) ) ;
#14878=CARTESIAN_POINT ( 'NONE',  ( 124.9522429225335998, -1091.716738251577226, -27.62619522811934658 ) ) ;
#14885=ORIENTED_EDGE ( 'NONE', *, *, #8236, .F. ) ;
#14888=CARTESIAN_POINT ( 'NONE',  ( -136.5850230665617460, -1073.277182683704496, -28.11073331261979291 ) ) ;
#14890=EDGE_LOOP ( 'NONE', ( #17605, #22006, #19740, #16626 ) ) ;
#14891=CARTESIAN_POINT ( 'NONE',  ( -135.6313030678082896, -1075.027834699371169, 32.48437713430732288 ) ) ;
#14897=AXIS2_PLACEMENT_3D ( 'NONE', #19554, #10170, #17515 ) ;
#14905=ORIENTED_EDGE ( 'NONE', *, *, #20929, .F. ) ;
#14906=CARTESIAN_POINT ( 'NONE',  ( -128.0900118278593141, 87.28149574061829696, 27.50000000000646594 ) ) ;
#14911=DIRECTION ( 'NONE',  ( 0.6964005597823107463, -0.7176533009294141507, 6.982962677686266711E-15 ) ) ;
#14914=DIRECTION ( 'NONE',  ( 0.000000000000000000, 0.000000000000000000, 1.000000000000000000 ) ) ;
#14915=ORIENTED_EDGE ( 'NONE', *, *, #11920, .T. ) ;
#14916=ADVANCED_FACE ( 'NONE', ( #19015 ), #15080, .F. ) ;
#14919=CARTESIAN_POINT ( 'NONE',  ( 132.4204480437716143, 80.55959301515268578, -27.62619522811937856 ) ) ;
#14929=ORIENTED_EDGE ( 'NONE', *, *, #21985, .F. ) ;
#14934=CARTESIAN_POINT ( 'NONE',  ( -175.1609685624536610, -1088.719770019218913, 27.50000000000675371 ) ) ;
#14938=CARTESIAN_POINT ( 'NONE',  ( 124.3723197571906240, -1092.501637924545548, -27.49999999999351274 ) ) ;
#14947=ADVANCED_FACE ( 'NONE', ( #2235 ), #12785, .F. ) ;
#14948=VERTEX_POINT ( 'NONE', #22644 ) ;
#14951=DIRECTION ( 'NONE',  ( -1.000000000000000000, 1.408839003528726857E-14, 6.982962677686266711E-15 ) ) ;
#14959=DIRECTION ( 'NONE',  ( -0.000000000000000000, -0.000000000000000000, -1.000000000000000000 ) ) ;
#14974=DIRECTION ( 'NONE',  ( -0.9423651898111408132, -0.3345860861306287348, 6.982962677686266711E-15 ) ) ;
#14975=VERTEX_POINT ( 'NONE', #22777 ) ;
#14978=EDGE_CURVE ( 'NONE', #17788, #14948, #782, .T. ) ;
#14988=ORIENTED_EDGE ( 'NONE', *, *, #22168, .T. ) ;
#15005=DIRECTION ( 'NONE',  ( -1.350636282998972974E-14, 0.000000000000000000, -1.000000000000000000 ) ) ;
#15007=ORIENTED_EDGE ( 'NONE', *, *, #1941, .F. ) ;
#15015=CONICAL_SURFACE ( 'NONE', #12021, 2.055000000000001492, 0.7853981633974633780 ) ;
#15023=EDGE_LOOP ( 'NONE', ( #9936, #7261 ) ) ;
#15028=EDGE_CURVE ( 'NONE', #5008, #590, #5991, .T. ) ;
#15029=FACE_OUTER_BOUND ( 'NONE', #7684, .T. ) ;
#15033=EDGE_LOOP ( 'NONE', ( #22794, #8219, #3149, #19139 ) ) ;
#15050=EDGE_CURVE ( 'NONE', #12140, #22609, #21217, .T. ) ;
#15065=ORIENTED_EDGE ( 'NONE', *, *, #22720, .F. ) ;
#15067=VECTOR ( 'NONE', #10131, 1000.000000000000000 ) ;
#15068=CARTESIAN_POINT ( 'NONE',  ( 123.9854850298561786, -1093.019475613610211, -27.62591505085370258 ) ) ;
#15071=CARTESIAN_POINT ( 'NONE',  ( 146.0000000000002274, -801.0618695410406644, -29.99999999999356604 ) ) ;
#15080=CONICAL_SURFACE ( 'NONE', #8909, 2.055000000000001492, 0.7853981633974633780 ) ;
#15089=DIRECTION ( 'NONE',  ( 0.9289202219288174023, 0.3702799228849934510, 6.982962677686266711E-15 ) ) ;
#15092=EDGE_LOOP ( 'NONE', ( #15990, #16924, #19388, #8749 ) ) ;
#15096=EDGE_CURVE ( 'NONE', #15482, #22916, #18, .T. ) ;
#15101=DIRECTION ( 'NONE',  ( 0.000000000000000000, -1.000000000000000000, 0.000000000000000000 ) ) ;
#15103=CYLINDRICAL_SURFACE ( 'NONE', #17081, 2.500000000000002220 ) ;
#15106=LINE ( 'NONE', #2511, #20707 ) ;
#15107=FACE_OUTER_BOUND ( 'NONE', #8660, .T. ) ;
#15113=CARTESIAN_POINT ( 'NONE',  ( -146.0000000000001421, -496.5240652294807546, 30.00000000000641620 ) ) ;
#15114=VERTEX_POINT ( 'NONE', #17462 ) ;
#15121=ORIENTED_EDGE ( 'NONE', *, *, #13600, .T. ) ;
#15122=ORIENTED_EDGE ( 'NONE', *, *, #21503, .F. ) ;
#15138=CARTESIAN_POINT ( 'NONE',  ( -146.0000000000005116, -784.4690652294799520, -29.99999999999356604 ) ) ;
#15140=LINE ( 'NONE', #22228, #23432 ) ;
#15141=ORIENTED_EDGE ( 'NONE', *, *, #20131, .T. ) ;
#15149=CARTESIAN_POINT ( 'NONE',  ( -128.5309343563513380, 86.63037569149894068, 27.75096515221181193 ) ) ;
#15163=ADVANCED_FACE ( 'NONE', ( #2943 ), #17690, .F. ) ;
#15183=FACE_OUTER_BOUND ( 'NONE', #15479, .T. ) ;
#15208=ORIENTED_EDGE ( 'NONE', *, *, #22126, .T. ) ;
#15220=DIRECTION ( 'NONE',  ( -1.000000000000000000, 1.408839003528726857E-14, 6.982962677686266711E-15 ) ) ;
#15224=CARTESIAN_POINT ( 'NONE',  ( -127.7157292285634753, 87.82777678213082595, 27.51597717546056998 ) ) ;
#15232=ORIENTED_EDGE ( 'NONE', *, *, #5004, .T. ) ;
#15244=EDGE_CURVE ( 'NONE', #17523, #6254, #12404, .T. ) ;
#15249=CARTESIAN_POINT ( 'NONE',  ( -136.3245111336061086, -1073.760768802671691, -32.24959887471651143 ) ) ;
#15260=FACE_OUTER_BOUND ( 'NONE', #5873, .T. ) ;
#15294=ORIENTED_EDGE ( 'NONE', *, *, #10080, .T. ) ;
#15303=CARTESIAN_POINT ( 'NONE',  ( -194.7500000000004832, -494.4690652294794404, -29.99999999999322498 ) ) ;
#15305=DIRECTION ( 'NONE',  ( -6.982962677686266711E-15, 0.000000000000000000, 1.000000000000000000 ) ) ;
#15317=ORIENTED_EDGE ( 'NONE', *, *, #2196, .F. ) ;
#15325=CIRCLE ( 'NONE', #4102, 2.055000000000001492 ) ;
#15343=CARTESIAN_POINT ( 'NONE',  ( -127.5319552722390739, 88.09441757049741284, 32.42079297023035878 ) ) ;
#15346=EDGE_CURVE ( 'NONE', #14427, #2037, #19109, .T. ) ;
#15347=VECTOR ( 'NONE', #16442, 1000.000000000000000 ) ;
#15348=EDGE_LOOP ( 'NONE', ( #3448, #3194 ) ) ;
#15351=ORIENTED_EDGE ( 'NONE', *, *, #13701, .F. ) ;
#15356=AXIS2_PLACEMENT_3D ( 'NONE', #12303, #3077, #802 ) ;
#15373=DIRECTION ( 'NONE',  ( -0.000000000000000000, -0.000000000000000000, -1.000000000000000000 ) ) ;
#15380=AXIS2_PLACEMENT_3D ( 'NONE', #2137, #20372, #9528 ) ;
#15388=VERTEX_POINT ( 'NONE', #19226 ) ;
#15390=( NAMED_UNIT ( * ) PLANE_ANGLE_UNIT ( ) SI_UNIT ( $, .RADIAN. ) );
#15397=CARTESIAN_POINT ( 'NONE',  ( 132.2605194320663600, 80.82189108482278073, -32.24903484778817386 ) ) ;
#15404=AXIS2_PLACEMENT_3D ( 'NONE', #19624, #1395, #3317 ) ;
#15406=CARTESIAN_POINT ( 'NONE',  ( 0.000000000000000000, -1000.000000000000000, -90.00000000000000000 ) ) ;
#15410=ORIENTED_EDGE ( 'NONE', *, *, #6374, .T. ) ;
#15419=VECTOR ( 'NONE', #6844, 1000.000000000000000 ) ;
#15425=CARTESIAN_POINT ( 'NONE',  ( -155.0000000000000284, -784.4690652294804067, 27.50000000000647660 ) ) ;
#15429=DIRECTION ( 'NONE',  ( -0.9423651898111408132, -0.3345860861306287348, 6.982962677686266711E-15 ) ) ;
#15439=ORIENTED_EDGE ( 'NONE', *, *, #1729, .T. ) ;
#15441=DIRECTION ( 'NONE',  ( 0.6964005597823107463, -0.7176533009294141507, 6.982962677686266711E-15 ) ) ;
#15465=AXIS2_PLACEMENT_3D ( 'NONE', #3188, #21565, #21679 ) ;
#15470=FACE_OUTER_BOUND ( 'NONE', #4480, .T. ) ;
#15479=EDGE_LOOP ( 'NONE', ( #950, #20525, #5113, #19595 ) ) ;
#15482=VERTEX_POINT ( 'NONE', #4742 ) ;
#15496=CARTESIAN_POINT ( 'NONE',  ( -146.4450000000005332, -204.4690652294800657, -32.49999999999356248 ) ) ;
#15507=UNCERTAINTY_MEASURE_WITH_UNIT (LENGTH_MEASURE( 1.000000000000000082E-05 ), #3325, 'distance_accuracy_value', 'NONE');
#15519=ORIENTED_EDGE ( 'NONE', *, *, #2838, .T. ) ;
#15530=CARTESIAN_POINT ( 'NONE',  ( 122.9560050114707934, -1094.375960373423595, 30.32918505548578381 ) ) ;
#15532=ORIENTED_EDGE ( 'NONE', *, *, #619, .F. ) ;
#15550=EDGE_LOOP ( 'NONE', ( #1411, #17964, #5998, #23463 ) ) ;
#15552=ADVANCED_FACE ( 'NONE', ( #16233 ), #6085, .F. ) ;
#15555=EDGE_LOOP ( 'NONE', ( #4862, #18953, #3390, #13240 ) ) ;
#15567=DIRECTION ( 'NONE',  ( -1.000000000000000000, 1.408839003528726857E-14, 6.982962677686266711E-15 ) ) ;
#15573=DIRECTION ( 'NONE',  ( -4.862939117679700002E-15, 5.011346215908450209E-15, 1.000000000000000000 ) ) ;
#15576=VERTEX_POINT ( 'NONE', #5340 ) ;
#15578=DIRECTION ( 'NONE',  ( 1.000000000000000000, -0.000000000000000000, -0.000000000000000000 ) ) ;
#15579=DIRECTION ( 'NONE',  ( 0.000000000000000000, 0.000000000000000000, -1.000000000000000000 ) ) ;
#15583=EDGE_CURVE ( 'NONE', #4214, #21432, #14188, .T. ) ;
#15584=EDGE_CURVE ( 'NONE', #12953, #13741, #10350, .T. ) ;
#15604=DIRECTION ( 'NONE',  ( 0.9289202219288174023, 0.3702799228849933955, 6.982962677686265922E-15 ) ) ;
#15606=ORIENTED_EDGE ( 'NONE', *, *, #5166, .F. ) ;
#15639=CARTESIAN_POINT ( 'NONE',  ( 126.3653543294811499, 77.28387428943223370, 30.00000000000641620 ) ) ;
#15640=AXIS2_PLACEMENT_3D ( 'NONE', #23280, #12355, #15829 ) ;
#15641=CARTESIAN_POINT ( 'NONE',  ( 145.9999999999998010, -801.0618695410399823, 30.00000000000641620 ) ) ;
#15646=LINE ( 'NONE', #17447, #8671 ) ;
#15663=PLANE ( 'NONE',  #6857 ) ;
#15673=DIRECTION ( 'NONE',  ( -1.000000000000000000, 1.408839003528726857E-14, 6.982962677686266711E-15 ) ) ;
#15674=FACE_OUTER_BOUND ( 'NONE', #12475, .T. ) ;
#15680=CARTESIAN_POINT ( 'NONE',  ( -145.0000000000000284, -1000.000000000000000, 90.00000000000000000 ) ) ;
#15687=EDGE_CURVE ( 'NONE', #14223, #15996, #2988, .T. ) ;
#15690=VERTEX_POINT ( 'NONE', #15496 ) ;
#15694=DIRECTION ( 'NONE',  ( -1.000000000000000000, 1.408839003528726857E-14, 6.982962677686266711E-15 ) ) ;
#15696=ORIENTED_EDGE ( 'NONE', *, *, #12405, .F. ) ;
#15697=CONICAL_SURFACE ( 'NONE', #2936, 2.055000000000001492, 0.7853981633974633780 ) ;
#15701=ORIENTED_EDGE ( 'NONE', *, *, #16399, .T. ) ;
#15702=CARTESIAN_POINT ( 'NONE',  ( -135.6291186032802614, -1075.032345129803616, -32.49999999999351274 ) ) ;
#15706=LINE ( 'NONE', #12231, #1296 ) ;
#15707=AXIS2_PLACEMENT_3D ( 'NONE', #12824, #20126, #3571 ) ;
#15715=CARTESIAN_POINT ( 'NONE',  ( 145.9999999999998010, -209.9999999999996874, 30.00000000000641620 ) ) ;
#15728=DIRECTION ( 'NONE',  ( 0.6964005597823107463, -0.7176533009294141507, 6.982962677686266711E-15 ) ) ;
#15753=AXIS2_PLACEMENT_3D ( 'NONE', #10123, #17467, #13881 ) ;
#15774=CIRCLE ( 'NONE', #21912, 2.055000000000001492 ) ;
#15775=DIRECTION ( 'NONE',  ( 0.000000000000000000, 0.000000000000000000, 1.000000000000000000 ) ) ;
#15781=VECTOR ( 'NONE', #12452, 1000.000000000000000 ) ;
#15786=DIRECTION ( 'NONE',  ( -2.775557561562891351E-17, 1.000000000000000000, -0.000000000000000000 ) ) ;
#15790=CARTESIAN_POINT ( 'NONE',  ( 131.8485914335931000, 81.49210221337234827, 28.34264858295340161 ) ) ;
#15791=VECTOR ( 'NONE', #12566, 1000.000000000000000 ) ;
#15794=CIRCLE ( 'NONE', #20789, 155.0000000000000284 ) ;
#15814=VECTOR ( 'NONE', #17786, 1000.000000000000114 ) ;
#15829=DIRECTION ( 'NONE',  ( -1.350636282998972974E-14, 0.000000000000000000, -1.000000000000000000 ) ) ;
#15830=ADVANCED_FACE ( 'NONE', ( #10631, #8802, #2543, #9934, #17852, #17970, #8565 ), #14379, .F. ) ;
#15851=AXIS2_PLACEMENT_3D ( 'NONE', #6261, #12330, #21339 ) ;
#15878=CARTESIAN_POINT ( 'NONE',  ( 126.7787238282401745, 77.44864885511553609, -32.49999999999356959 ) ) ;
#15882=EDGE_LOOP ( 'NONE', ( #20889, #23020 ) ) ;
#15889=VERTEX_POINT ( 'NONE', #7563 ) ;
#15898=LINE ( 'NONE', #23475, #12348 ) ;
#15907=CARTESIAN_POINT ( 'NONE',  ( -155.0000000000000284, 0.000000000000000000, 90.00000000000000000 ) ) ;
#15910=CARTESIAN_POINT ( 'NONE',  ( 131.6943452429968033, 81.74110354019241242, 28.74299381080684412 ) ) ;
#15914=FACE_OUTER_BOUND ( 'NONE', #2521, .T. ) ;
#15916=EDGE_CURVE ( 'NONE', #15388, #3131, #16880, .T. ) ;
#15920=FACE_OUTER_BOUND ( 'NONE', #21504, .T. ) ;
#15930=ORIENTED_EDGE ( 'NONE', *, *, #17472, .T. ) ;
#15933=ORIENTED_EDGE ( 'NONE', *, *, #21375, .F. ) ;
#15935=ADVANCED_FACE ( 'NONE', ( #5283 ), #10880, .F. ) ;
#15939=CARTESIAN_POINT ( 'NONE',  ( -134.8603954219446166, -1076.404761192049136, -31.65735141704661260 ) ) ;
#15947=LINE ( 'NONE', #14276, #4624 ) ;
#15953=VECTOR ( 'NONE', #14093, 1000.000000000000000 ) ;
#15958=VERTEX_POINT ( 'NONE', #17362 ) ;
#15966=CARTESIAN_POINT ( 'NONE',  ( -136.7463441837905975, -1072.975652424845066, 31.53022738271487313 ) ) ;
#15975=CARTESIAN_POINT ( 'NONE',  ( 124.4701338314433485, -1092.369831568443260, -27.49999999999351985 ) ) ;
#15979=LINE ( 'NONE', #3029, #8460 ) ;
#15983=ORIENTED_EDGE ( 'NONE', *, *, #107, .F. ) ;
#15990=ORIENTED_EDGE ( 'NONE', *, *, #12076, .F. ) ;
#15996=VERTEX_POINT ( 'NONE', #19019 ) ;
#15997=VECTOR ( 'NONE', #5858, 999.9999999999998863 ) ;
#16001=CARTESIAN_POINT ( 'NONE',  ( -122.8605704798723224, 82.74225173005862644, 27.94500000000642359 ) ) ;
#16011=CARTESIAN_POINT ( 'NONE',  ( -146.0000000000005116, -494.4690652294800657, -29.99999999999356604 ) ) ;
#16024=LINE ( 'NONE', #20971, #17769 ) ;
#16028=EDGE_LOOP ( 'NONE', ( #14385, #14032, #22801, #14162 ) ) ;
#16034=DIRECTION ( 'NONE',  ( -1.000000000000000000, -2.775557561562891351E-17, 0.000000000000000000 ) ) ;
#16035=CARTESIAN_POINT ( 'NONE',  ( 0.000000000000000000, -1000.000000000000000, 90.00000000000000000 ) ) ;
#16050=AXIS2_PLACEMENT_3D ( 'NONE', #20110, #13190, #12909 ) ;
#16053=CARTESIAN_POINT ( 'NONE',  ( 126.3653543294818178, 77.28387428943173632, -29.99999999999356604 ) ) ;
#16055=VERTEX_POINT ( 'NONE', #11591 ) ;
#16056=CARTESIAN_POINT ( 'NONE',  ( -135.1744136729190018, -1075.847854466910803, -32.17188107257633334 ) ) ;
#16068=AXIS2_PLACEMENT_3D ( 'NONE', #10200, #6436, #10457 ) ;
#16071=ADVANCED_FACE ( 'NONE', ( #5996 ), #22525, .F. ) ;
#16091=DIRECTION ( 'NONE',  ( 0.9423651898111409242, 0.3345860861306287903, -6.982962677686268288E-15 ) ) ;
#16094=CONICAL_SURFACE ( 'NONE', #4921, 2.055000000000001492, 0.7853981633974633780 ) ;
#16097=ORIENTED_EDGE ( 'NONE', *, *, #9748, .F. ) ;
#16103=EDGE_CURVE ( 'NONE', #18595, #9869, #1271, .T. ) ;
#16105=ORIENTED_EDGE ( 'NONE', *, *, #11100, .T. ) ;
#16108=ORIENTED_EDGE ( 'NONE', *, *, #6766, .F. ) ;
#16113=VECTOR ( 'NONE', #22460, 1000.000000000000114 ) ;
#16116=CARTESIAN_POINT ( 'NONE',  ( -129.3177328886526709, 85.45129583908980919, -29.83126738556711999 ) ) ;
#16120=CARTESIAN_POINT ( 'NONE',  ( 132.9260832389177267, 79.72254387118044860, 27.50000000000646239 ) ) ;
#16132=AXIS2_PLACEMENT_3D ( 'NONE', #3984, #11398, #18713 ) ;
#16152=LINE ( 'NONE', #1868, #15419 ) ;
#16156=CIRCLE ( 'NONE', #5351, 2.500000000000002220 ) ;
#16183=DIRECTION ( 'NONE',  ( -1.110223024625155594E-14, 0.000000000000000000, -1.000000000000000000 ) ) ;
#16184=ORIENTED_EDGE ( 'NONE', *, *, #8587, .F. ) ;
#16186=CARTESIAN_POINT ( 'NONE',  ( -146.0000000000005116, -204.4690652294800657, -29.99999999999356604 ) ) ;
#16193=CARTESIAN_POINT ( 'NONE',  ( -146.4450000000001069, -784.4690652294805204, 27.50000000000642331 ) ) ;
#16199=EDGE_LOOP ( 'NONE', ( #299, #14905, #12701, #22202 ) ) ;
#16200=EDGE_CURVE ( 'NONE', #404, #22916, #10488, .T. ) ;
#16202=EDGE_CURVE ( 'NONE', #21308, #11453, #10757, .T. ) ;
#16215=ORIENTED_EDGE ( 'NONE', *, *, #11100, .F. ) ;
#16229=VERTEX_POINT ( 'NONE', #6471 ) ;
#16233=FACE_OUTER_BOUND ( 'NONE', #14235, .T. ) ;
#16235=CARTESIAN_POINT ( 'NONE',  ( 146.4449999999997374, -209.9999999999996874, 32.50000000000641620 ) ) ;
#16240=VERTEX_POINT ( 'NONE', #20093 ) ;
#16242=PLANE ( 'NONE',  #8837 ) ;
#16243=DIRECTION ( 'NONE',  ( -0.9423651898111408132, -0.3345860861306287348, 6.982962677686266711E-15 ) ) ;
#16250=CARTESIAN_POINT ( 'NONE',  ( 133.4121500950858490, 78.90641005980415912, 32.24990070396069086 ) ) ;
#16252=ADVANCED_FACE ( 'NONE', ( #12190 ), #19265, .F. ) ;
#16265=CARTESIAN_POINT ( 'NONE',  ( 145.9999999999997726, -801.0618695410399823, 32.05500000000641592 ) ) ;
#16266=CARTESIAN_POINT ( 'NONE',  ( -146.0000000000005684, -786.5240652294799020, -29.99999999999356604 ) ) ;
#16270=DIRECTION ( 'NONE',  ( 1.000000000000000000, -0.000000000000000000, -0.000000000000000000 ) ) ;
#16277=CARTESIAN_POINT ( 'NONE',  ( 146.0000000000002558, -801.0618695410406644, -32.05499999999356930 ) ) ;
#16286=ADVANCED_FACE ( 'NONE', ( #7419 ), #8772, .F. ) ;
#16308=CARTESIAN_POINT ( 'NONE',  ( -127.7157292285630632, 87.82777678213136596, -32.48402282453940870 ) ) ;
#16315=EDGE_CURVE ( 'NONE', #15889, #1686, #16366, .T. ) ;
#16317=DIRECTION ( 'NONE',  ( -1.110223024625157172E-14, 0.000000000000000000, -1.000000000000000000 ) ) ;
#16321=ORIENTED_EDGE ( 'NONE', *, *, #7703, .F. ) ;
#16342=DIRECTION ( 'NONE',  ( -1.000000000000000000, 1.408839003528726857E-14, 6.982962677686266711E-15 ) ) ;
#16344=DIRECTION ( 'NONE',  ( 0.9423651898111409242, 0.3345860861306287903, -6.982962677686268288E-15 ) ) ;
#16355=DIRECTION ( 'NONE',  ( -1.110223024625157172E-14, 0.000000000000000000, -1.000000000000000000 ) ) ;
#16362=EDGE_CURVE ( 'NONE', #4214, #10971, #3689, .T. ) ;
#16366=LINE ( 'NONE', #10849, #1393 ) ;
#16369=VECTOR ( 'NONE', #11725, 1000.000000000000000 ) ;
#16379=ORIENTED_EDGE ( 'NONE', *, *, #15916, .F. ) ;
#16380=CARTESIAN_POINT ( 'NONE',  ( 123.1031131805784469, -1094.184009126531237, -31.11320915316581193 ) ) ;
#16386=ORIENTED_EDGE ( 'NONE', *, *, #21802, .T. ) ;
#16399=EDGE_CURVE ( 'NONE', #493, #12317, #3547, .T. ) ;
#16400=DIRECTION ( 'NONE',  ( -0.7071067811865320296, 9.875400524328840493E-15, 0.7071067811865631159 ) ) ;
#16402=CONICAL_SURFACE ( 'NONE', #6383, 2.055000000000001492, 0.7853981633974633780 ) ;
#16403=DIRECTION ( 'NONE',  ( -1.350636282998972974E-14, 0.000000000000000000, -1.000000000000000000 ) ) ;
#16412=DIRECTION ( 'NONE',  ( 0.000000000000000000, 0.000000000000000000, -1.000000000000000000 ) ) ;
#16414=VERTEX_POINT ( 'NONE', #22615 ) ;
#16418=CARTESIAN_POINT ( 'NONE',  ( -127.5319552722386760, 88.09441757049788180, -27.57920702976963767 ) ) ;
#16442=DIRECTION ( 'NONE',  ( -2.775557561562891351E-17, 1.000000000000000000, -0.000000000000000000 ) ) ;
#16450=EDGE_LOOP ( 'NONE', ( #13620, #1787, #8682, #2565 ) ) ;
#16463=CIRCLE ( 'NONE', #277, 2.499999999999998668 ) ;
#16464=CARTESIAN_POINT ( 'NONE',  ( -129.2813770747755484, 85.50638651248962674, 29.34395718620176297 ) ) ;
#16491=CARTESIAN_POINT ( 'NONE',  ( 124.3711180590059229, -1092.503257236082163, -32.49999999999351985 ) ) ;
#16493=DIRECTION ( 'NONE',  ( -0.7232617928448825673, 0.6905739489807055653, 6.982962677686266711E-15 ) ) ;
#16503=CYLINDRICAL_SURFACE ( 'NONE', #21112, 2.500000000000002220 ) ;
#16523=CARTESIAN_POINT ( 'NONE',  ( -136.6968504244148335, -1073.068359172759074, 31.65640384616915526 ) ) ;
#16524=DIRECTION ( 'NONE',  ( 1.000000000000000000, -0.000000000000000000, -0.000000000000000000 ) ) ;
#16529=CARTESIAN_POINT ( 'NONE',  ( -126.7581711459445160, 89.20411804604358963, -31.53250949154612925 ) ) ;
#16532=FACE_BOUND ( 'NONE', #22565, .T. ) ;
#16536=CIRCLE ( 'NONE', #19603, 2.055000000000001492 ) ;
#16547=ORIENTED_EDGE ( 'NONE', *, *, #11925, .F. ) ;
#16548=PRODUCT_DEFINITION_SHAPE ( 'NONE', 'NONE',  #11555 ) ;
#16555=ORIENTED_EDGE ( 'NONE', *, *, #23209, .F. ) ;
#16560=ADVANCED_FACE ( 'NONE', ( #8153 ), #19501, .F. ) ;
#16563=CARTESIAN_POINT ( 'NONE',  ( 125.9168667295997892, -1090.387741168242883, -29.34624901867154634 ) ) ;
#16570=EDGE_CURVE ( 'NONE', #19928, #22176, #19125, .T. ) ;
#16593=CARTESIAN_POINT ( 'NONE',  ( 124.8644691973863701, -1091.836575763269366, 27.56549073392524818 ) ) ;
#16599=CARTESIAN_POINT ( 'NONE',  ( 134.0610795706241447, 77.79865694966419198, 30.80845853161018155 ) ) ;
#16603=ADVANCED_FACE ( 'NONE', ( #19112 ), #21297, .F. ) ;
#16615=DIRECTION ( 'NONE',  ( 1.000000000000000000, -0.000000000000000000, 6.982962677686266711E-15 ) ) ;
#16625=CARTESIAN_POINT ( 'NONE',  ( 146.4449999999997658, -209.9999999999996874, 30.00000000000641975 ) ) ;
#16626=ORIENTED_EDGE ( 'NONE', *, *, #12166, .T. ) ;
#16628=CARTESIAN_POINT ( 'NONE',  ( 123.2631315123078366, -1093.974511992577163, -28.46977261728505937 ) ) ;
#16640=ADVANCED_FACE ( 'NONE', ( #1706 ), #23451, .F. ) ;
#16644=ORIENTED_EDGE ( 'NONE', *, *, #8640, .F. ) ;
#16652=LINE ( 'NONE', #7576, #21755 ) ;
#16653=VERTEX_POINT ( 'NONE', #16235 ) ;
#16654=ORIENTED_EDGE ( 'NONE', *, *, #21682, .T. ) ;
#16656=CARTESIAN_POINT ( 'NONE',  ( -127.2684398464540863, 88.47467185906484133, -27.75009929603929493 ) ) ;
#16666=PLANE ( 'NONE',  #10307 ) ;
#16667=ORIENTED_EDGE ( 'NONE', *, *, #6658, .T. ) ;
#16681=CARTESIAN_POINT ( 'NONE',  ( 125.7677891478055301, -1090.595098045220993, -31.25700618919319851 ) ) ;
#16705=EDGE_CURVE ( 'NONE', #22268, #19341, #21463, .T. ) ;
#16707=CARTESIAN_POINT ( 'NONE',  ( 125.9551925347493722, -1090.334326554368772, 30.33200430454450114 ) ) ;
#16713=DIRECTION ( 'NONE',  ( 1.000000000000000000, -0.000000000000000000, -0.000000000000000000 ) ) ;
#16719=CARTESIAN_POINT ( 'NONE',  ( 131.8501689178089293, 81.48954978393982174, -28.33934113061009086 ) ) ;
#16739=DIRECTION ( 'NONE',  ( -1.110223024625155594E-14, 0.000000000000000000, -1.000000000000000000 ) ) ;
#16745=DIRECTION ( 'NONE',  ( -1.350636282998972974E-14, 0.000000000000000000, -1.000000000000000000 ) ) ;
#16752=ORIENTED_EDGE ( 'NONE', *, *, #6902, .T. ) ;
#16772=DIRECTION ( 'NONE',  ( -0.7071067811865416886, 9.961996129952529179E-15, -0.7071067811865532349 ) ) ;
#16788=CARTESIAN_POINT ( 'NONE',  ( -146.0000000000000853, -204.4690652294807478, 30.00000000000641620 ) ) ;
#16792=CARTESIAN_POINT ( 'NONE',  ( 125.8877979345642615, -1090.428239381491721, -29.18615827854500822 ) ) ;
#16803=CARTESIAN_POINT ( 'NONE',  ( -135.9487776228375253, -1074.451030117129676, -27.51610016701187078 ) ) ;
#16809=DIRECTION ( 'NONE',  ( -1.000000000000000000, 1.408839003528726857E-14, 6.982962677686266711E-15 ) ) ;
#16810=ORIENTED_EDGE ( 'NONE', *, *, #18027, .T. ) ;
#16815=AXIS2_PLACEMENT_3D ( 'NONE', #13242, #3997, #11902 ) ;
#16816=CARTESIAN_POINT ( 'NONE',  ( 125.9265396616754629, -1090.374350352354213, 29.34395718620176297 ) ) ;
#16820=DIRECTION ( 'NONE',  ( -1.000000000000000000, 1.408839003528726857E-14, 6.982962677686266711E-15 ) ) ;
#16833=CARTESIAN_POINT ( 'NONE',  ( 132.7558223547129046, 80.00574117445245292, -27.49999999999351630 ) ) ;
#16838=CIRCLE ( 'NONE', #18001, 155.0000000000000284 ) ;
#16840=CARTESIAN_POINT ( 'NONE',  ( 146.0000000000002558, -210.0000000000003411, -32.05499999999356930 ) ) ;
#16843=ORIENTED_EDGE ( 'NONE', *, *, #23653, .T. ) ;
#16854=VECTOR ( 'NONE', #16772, 1000.000000000000114 ) ;
#16864=EDGE_CURVE ( 'NONE', #12773, #15576, #13449, .T. ) ;
#16865=ADVANCED_FACE ( 'NONE', ( #13344 ), #12646, .F. ) ;
#16866=CARTESIAN_POINT ( 'NONE',  ( 155.0000000000000284, -210.0000000000003411, -29.99999999999350564 ) ) ;
#16877=AXIS2_PLACEMENT_3D ( 'NONE', #22095, #5566, #23441 ) ;
#16879=CYLINDRICAL_SURFACE ( 'NONE', #11166, 2.500000000000002220 ) ;
#16880=CIRCLE ( 'NONE', #8402, 2.055000000000001492 ) ;
#16887=ORIENTED_EDGE ( 'NONE', *, *, #8157, .T. ) ;
#16896=LINE ( 'NONE', #22320, #13761 ) ;
#16899=CARTESIAN_POINT ( 'NONE',  ( -127.4422799395779009, 88.22408193900459139, 27.62610291900639581 ) ) ;
#16907=CARTESIAN_POINT ( 'NONE',  ( -129.1311602790084123, 85.73302760282720669, -31.25700618919315232 ) ) ;
#16920=DIRECTION ( 'NONE',  ( 1.000000000000000000, -0.000000000000000000, 6.982962677686266711E-15 ) ) ;
#16924=ORIENTED_EDGE ( 'NONE', *, *, #19053, .F. ) ;
#16926=LINE ( 'NONE', #22353, #13563 ) ;
#16930=VECTOR ( 'NONE', #19004, 1000.000000000000000 ) ;
#16931=CARTESIAN_POINT ( 'NONE',  ( -135.1744136729186039, -1075.847854466910576, 27.82811892742367021 ) ) ;
#16935=AXIS2_PLACEMENT_3D ( 'NONE', #8557, #8925, #21342 ) ;
#16955=AXIS2_PLACEMENT_3D ( 'NONE', #74, #189, #14700 ) ;
#16957=CIRCLE ( 'NONE', #13543, 2.055000000000001492 ) ;
#16961=CARTESIAN_POINT ( 'NONE',  ( 132.8404720734533555, 79.86494211668889420, -27.49999999999351985 ) ) ;
#16992=DIRECTION ( 'NONE',  ( -1.000000000000000000, 1.408839003528726857E-14, 6.982962677686266711E-15 ) ) ;
#16995=ORIENTED_EDGE ( 'NONE', *, *, #19411, .F. ) ;
#17011=CARTESIAN_POINT ( 'NONE',  ( 146.4450000000002490, -801.0618695410406644, -29.99999999999356248 ) ) ;
#17012=EDGE_CURVE ( 'NONE', #11094, #2904, #16838, .T. ) ;
#17038=LINE ( 'NONE', #11753, #7715 ) ;
#17045=FACE_OUTER_BOUND ( 'NONE', #11893, .T. ) ;
#17052=CARTESIAN_POINT ( 'NONE',  ( -136.7463441837909386, -1072.975652424845066, -28.46977261728502384 ) ) ;
#17055=CARTESIAN_POINT ( 'NONE',  ( -134.9759958199650782, -1076.200356551567666, 28.11255663403409244 ) ) ;
#17062=VERTEX_POINT ( 'NONE', #17999 ) ;
#17064=EDGE_LOOP ( 'NONE', ( #6683, #18403, #392, #18978 ) ) ;
#17072=( NAMED_UNIT ( * ) SI_UNIT ( $, .STERADIAN. ) SOLID_ANGLE_UNIT ( ) );
#17081=AXIS2_PLACEMENT_3D ( 'NONE', #7583, #14974, #20736 ) ;
#17084=CARTESIAN_POINT ( 'NONE',  ( 122.9460700935429003, -1094.388896850126912, 29.67072815018520515 ) ) ;
#17088=FACE_BOUND ( 'NONE', #3222, .T. ) ;
#17098=DIRECTION ( 'NONE',  ( 6.753181414994864868E-15, 0.000000000000000000, -1.000000000000000000 ) ) ;
#17105=ORIENTED_EDGE ( 'NONE', *, *, #11341, .T. ) ;
#17109=VERTEX_POINT ( 'NONE', #23424 ) ;
#17128=CARTESIAN_POINT ( 'NONE',  ( 132.8404720734530144, 79.86494211668951948, 32.50000000000646594 ) ) ;
#17131=EDGE_CURVE ( 'NONE', #6254, #13113, #6886, .T. ) ;
#17141=CARTESIAN_POINT ( 'NONE',  ( -127.0280029979308267, 88.81950979153417336, 28.00660068667234626 ) ) ;
#17142=EDGE_CURVE ( 'NONE', #10971, #4214, #19534, .T. ) ;
#17152=CARTESIAN_POINT ( 'NONE',  ( -155.0000000000000284, -494.4690652294800088, -27.49999999999350209 ) ) ;
#17164=CARTESIAN_POINT ( 'NONE',  ( -135.7895026000616951, -1074.740959209979792, -32.49999999999351985 ) ) ;
#17169=CARTESIAN_POINT ( 'NONE',  ( -135.4687158836533456, -1075.321440059930865, 27.56549073392519844 ) ) ;
#17176=ORIENTED_EDGE ( 'NONE', *, *, #9452, .F. ) ;
#17186=FACE_BOUND ( 'NONE', #22835, .T. ) ;
#17187=AXIS2_PLACEMENT_3D ( 'NONE', #19919, #8956, #16317 ) ;
#17198=CARTESIAN_POINT ( 'NONE',  ( 131.5246926503486975, 82.01375679560341325, -29.66799569545553439 ) ) ;
#17207=CARTESIAN_POINT ( 'NONE',  ( 123.3278826340506953, -1093.889547229275422, 28.34183984639747322 ) ) ;
#17215=CARTESIAN_POINT ( 'NONE',  ( 155.0000000000000284, 2.775557561562891351E-16, -90.00000000000000000 ) ) ;
#17217=CARTESIAN_POINT ( 'NONE',  ( -129.6400180686265173, -1072.557589128678728, 27.50000000000641975 ) ) ;
#17245=ADVANCED_FACE ( 'NONE', ( #20624 ), #16666, .F. ) ;
#17246=CARTESIAN_POINT ( 'NONE',  ( -155.0000000000000284, -1000.000000000000000, 90.00000000000000000 ) ) ;
#17263=EDGE_CURVE ( 'NONE', #16229, #6064, #120, .T. ) ;
#17276=EDGE_CURVE ( 'NONE', #13152, #4047, #7653, .T. ) ;
#17282=CARTESIAN_POINT ( 'NONE',  ( 146.4450000000002206, -210.0000000000003411, -29.99999999999356248 ) ) ;
#17287=VECTOR ( 'NONE', #6616, 1000.000000000000114 ) ;
#17295=CARTESIAN_POINT ( 'NONE',  ( 145.0000000000000284, -500.0000000000000000, -27.49999999999996803 ) ) ;
#17306=ADVANCED_FACE ( 'NONE', ( #21246 ), #2519, .F. ) ;
#17315=ORIENTED_EDGE ( 'NONE', *, *, #3129, .F. ) ;
#17322=VECTOR ( 'NONE', #4038, 1000.000000000000000 ) ;
#17362=CARTESIAN_POINT ( 'NONE',  ( -155.0000000000000284, -204.4690652294806057, 27.50000000000647660 ) ) ;
#17369=CARTESIAN_POINT ( 'NONE',  ( 132.6690927018904347, 80.14999981558261766, 27.50000000000646594 ) ) ;
#17387=EDGE_LOOP ( 'NONE', ( #10692, #16995, #22114, #455 ) ) ;
#17396=CARTESIAN_POINT ( 'NONE',  ( -134.8072682999804499, -1076.498424757946623, -31.52881987646421891 ) ) ;
#17409=EDGE_CURVE ( 'NONE', #5229, #21974, #16463, .T. ) ;
#17410=EDGE_LOOP ( 'NONE', ( #14185, #8165, #1066, #15532 ) ) ;
#17415=CYLINDRICAL_SURFACE ( 'NONE', #21011, 145.0000000000000284 ) ;
#17420=DIRECTION ( 'NONE',  ( -1.110223024625157172E-14, 0.000000000000000000, -1.000000000000000000 ) ) ;
#17428=DIRECTION ( 'NONE',  ( -1.110223024625157172E-14, 0.000000000000000000, -1.000000000000000000 ) ) ;
#17440=CARTESIAN_POINT ( 'NONE',  ( -129.6400180686270858, -1072.557589128678273, -27.49999999999356248 ) ) ;
#17445=CARTESIAN_POINT ( 'NONE',  ( 123.5484583266988068, -1093.599130927304714, 28.00660068667236757 ) ) ;
#17447=CARTESIAN_POINT ( 'NONE',  ( 153.5653415408403646, -1122.352966361445169, 27.50000000000675371 ) ) ;
#17449=DIRECTION ( 'NONE',  ( 2.775557561562891351E-17, -1.000000000000000000, 0.000000000000000000 ) ) ;
#17453=ORIENTED_EDGE ( 'NONE', *, *, #6248, .T. ) ;
#17458=LINE ( 'NONE', #11582, #5384 ) ;
#17462=CARTESIAN_POINT ( 'NONE',  ( -122.8605704798722940, 82.74225173005859801, 32.05500000000642302 ) ) ;
#17465=ORIENTED_EDGE ( 'NONE', *, *, #17409, .F. ) ;
#17467=DIRECTION ( 'NONE',  ( -0.7232617928448825673, 0.6905739489807055653, 6.982962677686266711E-15 ) ) ;
#17472=EDGE_CURVE ( 'NONE', #14975, #8155, #5287, .T. ) ;
#17477=CARTESIAN_POINT ( 'NONE',  ( -146.0000000000001137, -784.4690652294805204, 27.94500000000641649 ) ) ;
#17479=CARTESIAN_POINT ( 'NONE',  ( -194.7500000000004832, -784.4690652294792699, -29.99999999999322498 ) ) ;
#17485=EDGE_LOOP ( 'NONE', ( #11543, #6593 ) ) ;
#17487=CARTESIAN_POINT ( 'NONE',  ( -194.7500000000000568, -784.4690652294799520, 27.50000000000675371 ) ) ;
#17493=CARTESIAN_POINT ( 'NONE',  ( -126.6052862049310619, 89.42094583968740551, 28.88679084683406373 ) ) ;
#17495=CARTESIAN_POINT ( 'NONE',  ( -135.0351526491288041, -1076.095746396249297, -27.99555145635498477 ) ) ;
#17498=DIRECTION ( 'NONE',  ( 0.000000000000000000, 0.000000000000000000, 1.000000000000000000 ) ) ;
#17501=CARTESIAN_POINT ( 'NONE',  ( 132.8404720734533555, 79.86494211668889420, -27.49999999999351985 ) ) ;
#17505=CARTESIAN_POINT ( 'NONE',  ( -158.1195828810603246, 116.4077317428679947, 30.00000000000675726 ) ) ;
#17509=ADVANCED_FACE ( 'NONE', ( #1304 ), #16094, .F. ) ;
#17511=AXIS2_PLACEMENT_3D ( 'NONE', #4681, #8419, #11846 ) ;
#17515=DIRECTION ( 'NONE',  ( 0.000000000000000000, 0.000000000000000000, -1.000000000000000000 ) ) ;
#17520=DIRECTION ( 'NONE',  ( 0.000000000000000000, 0.000000000000000000, -1.000000000000000000 ) ) ;
#17523=VERTEX_POINT ( 'NONE', #7783 ) ;
#17535=ORIENTED_EDGE ( 'NONE', *, *, #2203, .F. ) ;
#17539=CARTESIAN_POINT ( 'NONE',  ( 132.6690927018907473, 80.14999981558196396, -32.49999999999350564 ) ) ;
#17546=CIRCLE ( 'NONE', #15640, 2.055000000000001492 ) ;
#17550=EDGE_LOOP ( 'NONE', ( #17936, #5175, #15208, #854 ) ) ;
#17551=AXIS2_PLACEMENT_3D ( 'NONE', #5179, #7428, #12481 ) ;
#17552=CARTESIAN_POINT ( 'NONE',  ( -146.0000000000005116, -204.4690652294800657, -29.99999999999356604 ) ) ;
#17579=AXIS2_PLACEMENT_3D ( 'NONE', #3435, #5606, #22135 ) ;
#17581=DIRECTION ( 'NONE',  ( -1.350636282998972974E-14, 0.000000000000000000, -1.000000000000000000 ) ) ;
#17588=ORIENTED_EDGE ( 'NONE', *, *, #15050, .T. ) ;
#17589=DIRECTION ( 'NONE',  ( 0.000000000000000000, -1.000000000000000000, 0.000000000000000000 ) ) ;
#17593=PLANE ( 'NONE',  #2655 ) ;
#17597=EDGE_LOOP ( 'NONE', ( #9162, #19250, #20299, #13441 ) ) ;
#17605=ORIENTED_EDGE ( 'NONE', *, *, #11972, .F. ) ;
#17606=LINE ( 'NONE', #4457, #9430 ) ;
#17607=CARTESIAN_POINT ( 'NONE',  ( -126.6511612778954685, 89.35598455390400829, 28.74044610054854942 ) ) ;
#17609=CARTESIAN_POINT ( 'NONE',  ( -135.7895026000616951, -1074.740959209979792, -32.49999999999351985 ) ) ;
#17611=ORIENTED_EDGE ( 'NONE', *, *, #22876, .F. ) ;
#17617=CARTESIAN_POINT ( 'NONE',  ( 133.1749347183809675, 79.30613235828936070, -32.42132972170174554 ) ) ;
#17620=CARTESIAN_POINT ( 'NONE',  ( -146.4450000000000500, -494.4690652294806910, 32.50000000000641620 ) ) ;
#17636=CARTESIAN_POINT ( 'NONE',  ( -155.0000000000000284, -204.4690652294806625, 32.50000000000648015 ) ) ;
#17646=CARTESIAN_POINT ( 'NONE',  ( -129.2206655591611764, -1072.408698320350140, -27.94499999999358053 ) ) ;
#17649=CYLINDRICAL_SURFACE ( 'NONE', #3816, 2.500000000000002220 ) ;
#17655=DIRECTION ( 'NONE',  ( -0.9423651898111408132, -0.3345860861306287348, 6.982962677686266711E-15 ) ) ;
#17656=CARTESIAN_POINT ( 'NONE',  ( 132.4977819882884660, 80.43276747726498854, -32.43450926607475537 ) ) ;
#17660=DIRECTION ( 'NONE',  ( 1.110223024625155594E-14, 0.000000000000000000, -1.000000000000000000 ) ) ;
#17683=FACE_OUTER_BOUND ( 'NONE', #14425, .T. ) ;
#17690=PLANE ( 'NONE',  #9665 ) ;
#17696=ADVANCED_FACE ( 'NONE', ( #23336 ), #20727, .F. ) ;
#17701=CIRCLE ( 'NONE', #1882, 2.499999999999998668 ) ;
#17706=AXIS2_PLACEMENT_3D ( 'NONE', #2623, #8079, #11619 ) ;
#17711=CARTESIAN_POINT ( 'NONE',  ( 171.6502151485116201, 95.33502053007514121, -27.49999999999322498 ) ) ;
#17720=LINE ( 'NONE', #21698, #9218 ) ;
#17724=ORIENTED_EDGE ( 'NONE', *, *, #5882, .F. ) ;
#17729=AXIS2_PLACEMENT_3D ( 'NONE', #3426, #12653, #3302 ) ;
#17732=CIRCLE ( 'NONE', #6559, 2.499999999999998668 ) ;
#17734=AXIS2_PLACEMENT_3D ( 'NONE', #3447, #19630, #10608 ) ;
#17745=CARTESIAN_POINT ( 'NONE',  ( -134.6768122279369209, -1076.727833257003113, -31.11299551804361130 ) ) ;
#17756=CIRCLE ( 'NONE', #7331, 2.055000000000001492 ) ;
#17759=CARTESIAN_POINT ( 'NONE',  ( -155.0000000000000284, -204.4690652294800088, -27.49999999999350209 ) ) ;
#17769=VECTOR ( 'NONE', #15673, 1000.000000000000000 ) ;
#17774=ORIENTED_EDGE ( 'NONE', *, *, #11070, .F. ) ;
#17779=CARTESIAN_POINT ( 'NONE',  ( -136.8702482660834789, -1072.742966597998702, 28.88679084683412768 ) ) ;
#17786=DIRECTION ( 'NONE',  ( 0.4924295582441687857, -0.5074575156280874966, 0.7071067811865630048 ) ) ;
#17788=VERTEX_POINT ( 'NONE', #17440 ) ;
#17807=EDGE_LOOP ( 'NONE', ( #6112, #23159, #22564, #13950 ) ) ;
#17809=LINE ( 'NONE', #14204, #1367 ) ;
#17817=ORIENTED_EDGE ( 'NONE', *, *, #17012, .T. ) ;
#17843=FACE_OUTER_BOUND ( 'NONE', #23198, .T. ) ;
#17852=FACE_BOUND ( 'NONE', #23755, .T. ) ;
#17862=EDGE_LOOP ( 'NONE', ( #15141, #14477 ) ) ;
#17864=CARTESIAN_POINT ( 'NONE',  ( 133.6917068022189596, 78.43176171823509435, -31.88829724122658504 ) ) ;
#17874=AXIS2_PLACEMENT_3D ( 'NONE', #16011, #10115, #21076 ) ;
#17921=DIRECTION ( 'NONE',  ( -0.000000000000000000, -1.000000000000000000, -0.000000000000000000 ) ) ;
#17927=CIRCLE ( 'NONE', #18676, 2.499999999999946709 ) ;
#17932=VERTEX_POINT ( 'NONE', #12874 ) ;
#17936=ORIENTED_EDGE ( 'NONE', *, *, #6095, .F. ) ;
#17939=ADVANCED_FACE ( 'NONE', ( #23457 ), #14426, .F. ) ;
#17940=CARTESIAN_POINT ( 'NONE',  ( -155.0000000000000284, -1000.000000000000000, 90.00000000000000000 ) ) ;
#17957=DIRECTION ( 'NONE',  ( -6.753181414994864868E-15, 6.753181414994864868E-15, -1.000000000000000000 ) ) ;
#17964=ORIENTED_EDGE ( 'NONE', *, *, #15584, .F. ) ;
#17967=DIRECTION ( 'NONE',  ( -1.000000000000000000, 1.408839003528726857E-14, 6.982962677686266711E-15 ) ) ;
#17969=DIRECTION ( 'NONE',  ( -1.000000000000000000, 0.000000000000000000, 0.000000000000000000 ) ) ;
#17970=FACE_BOUND ( 'NONE', #6265, .T. ) ;
#17971=EDGE_CURVE ( 'NONE', #8260, #4200, #3402, .T. ) ;
#17993=DIRECTION ( 'NONE',  ( -1.000000000000000000, 1.408839003528726857E-14, 6.982962677686266711E-15 ) ) ;
#17999=CARTESIAN_POINT ( 'NONE',  ( 124.4701338314437891, -1092.369831568442805, 27.50000000000646239 ) ) ;
#18001=AXIS2_PLACEMENT_3D ( 'NONE', #23661, #5198, #19803 ) ;
#18016=FACE_OUTER_BOUND ( 'NONE', #11825, .T. ) ;
#18017=VERTEX_POINT ( 'NONE', #7506 ) ;
#18027=EDGE_CURVE ( 'NONE', #45, #2904, #15140, .T. ) ;
#18033=EDGE_CURVE ( 'NONE', #22609, #4934, #22716, .T. ) ;
#18046=CARTESIAN_POINT ( 'NONE',  ( 133.8630869304073485, 78.13886732029855864, 28.46749050845387075 ) ) ;
#18055=CARTESIAN_POINT ( 'NONE',  ( 125.6044290879524965, 79.19280534549594108, 30.00000000000641620 ) ) ;
#18058=VECTOR ( 'NONE', #15786, 1000.000000000000000 ) ;
#18064=EDGE_LOOP ( 'NONE', ( #14471, #4719, #8586, #10597 ) ) ;
#18070=ADVANCED_FACE ( 'NONE', ( #11404 ), #22659, .F. ) ;
#18076=EDGE_CURVE ( 'NONE', #2426, #1928, #6863, .T. ) ;
#18095=VECTOR ( 'NONE', #8309, 1000.000000000000000 ) ;
#18106=DIRECTION ( 'NONE',  ( -1.000000000000000000, 1.408839003528726857E-14, 6.982962677686266711E-15 ) ) ;
#18117=FACE_BOUND ( 'NONE', #2424, .T. ) ;
#18126=( GEOMETRIC_REPRESENTATION_CONTEXT ( 3 ) GLOBAL_UNCERTAINTY_ASSIGNED_CONTEXT ( ( #9655 ) ) GLOBAL_UNIT_ASSIGNED_CONTEXT ( ( #11540, #5954, #17072 ) ) REPRESENTATION_CONTEXT ( 'NONE', 'WORKASPACE' ) );
#18132=ORIENTED_EDGE ( 'NONE', *, *, #18779, .F. ) ;
#18140=CARTESIAN_POINT ( 'NONE',  ( 125.3835310783082093, -1091.126227143374990, -31.99040335529153367 ) ) ;
#18142=ORIENTED_EDGE ( 'NONE', *, *, #1862, .F. ) ;
#18151=FACE_OUTER_BOUND ( 'NONE', #1070, .T. ) ;
#18154=DIRECTION ( 'NONE',  ( 0.000000000000000000, 0.000000000000000000, -1.000000000000000000 ) ) ;
#18155=CARTESIAN_POINT ( 'NONE',  ( -194.7500000000000000, -204.4690652294800657, 32.50000000000675726 ) ) ;
#18159=DIRECTION ( 'NONE',  ( -1.110223024625157172E-14, 0.000000000000000000, -1.000000000000000000 ) ) ;
#18163=EDGE_LOOP ( 'NONE', ( #18175, #19493, #9151, #16810 ) ) ;
#18165=CARTESIAN_POINT ( 'NONE',  ( 134.1263161626745557, 77.68610759098336871, 30.16266818053253118 ) ) ;
#18175=ORIENTED_EDGE ( 'NONE', *, *, #790, .T. ) ;
#18186=EDGE_LOOP ( 'NONE', ( #22083, #242, #7955, #11737 ) ) ;
#18190=EDGE_LOOP ( 'NONE', ( #13626, #21256 ) ) ;
#18194=CARTESIAN_POINT ( 'NONE',  ( -146.4450000000005332, -494.4690652294800657, -32.49999999999356248 ) ) ;
#18202=CARTESIAN_POINT ( 'NONE',  ( -194.7500000000004547, -204.4690652294793836, -27.49999999999322498 ) ) ;
#18216=CYLINDRICAL_SURFACE ( 'NONE', #10587, 2.500000000000002220 ) ;
#18217=ORIENTED_EDGE ( 'NONE', *, *, #19775, .F. ) ;
#18222=CARTESIAN_POINT ( 'NONE',  ( -127.0280029979305141, 88.81950979153471337, -31.99339931332765374 ) ) ;
#18228=DIRECTION ( 'NONE',  ( 5.551115123125785858E-15, 0.000000000000000000, -1.000000000000000000 ) ) ;
#18238=AXIS2_PLACEMENT_3D ( 'NONE', #19607, #1013, #8392 ) ;
#18241=ORIENTED_EDGE ( 'NONE', *, *, #19198, .T. ) ;
#18244=ADVANCED_FACE ( 'NONE', ( #13426 ), #16402, .F. ) ;
#18259=EDGE_CURVE ( 'NONE', #9588, #4934, #19874, .T. ) ;
#18279=CARTESIAN_POINT ( 'NONE',  ( 155.0000000000000284, 2.775557561562891351E-16, 90.00000000000000000 ) ) ;
#18287=ADVANCED_FACE ( 'NONE', ( #15107 ), #23334, .F. ) ;
#18294=CARTESIAN_POINT ( 'NONE',  ( 123.4701789281957787, -1093.702342252440303, -28.11073331261971830 ) ) ;
#18306=CIRCLE ( 'NONE', #20611, 2.055000000000001492 ) ;
#18314=EDGE_CURVE ( 'NONE', #10087, #18017, #12970, .T. ) ;
#18316=CYLINDRICAL_SURFACE ( 'NONE', #14488, 2.500000000000002220 ) ;
#18321=DIRECTION ( 'NONE',  ( 1.000000000000000000, 0.000000000000000000, -0.000000000000000000 ) ) ;
#18324=FACE_OUTER_BOUND ( 'NONE', #5206, .T. ) ;
#18344=EDGE_LOOP ( 'NONE', ( #13803, #4965, #17724, #15007 ) ) ;
#18346=VECTOR ( 'NONE', #2205, 1000.000000000000000 ) ;
#18360=ORIENTED_EDGE ( 'NONE', *, *, #5004, .F. ) ;
#18363=CYLINDRICAL_SURFACE ( 'NONE', #18881, 2.500000000000002220 ) ;
#18371=DIRECTION ( 'NONE',  ( 0.6964005597823107463, -0.7176533009294141507, 6.982962677686266711E-15 ) ) ;
#18375=CARTESIAN_POINT ( 'NONE',  ( 125.2206635291107943, -1091.349901830162025, 27.82811892742366311 ) ) ;
#18377=AXIS2_PLACEMENT_3D ( 'NONE', #12960, #7367, #22198 ) ;
#18379=CARTESIAN_POINT ( 'NONE',  ( 134.0852850658430384, 77.75691219176937352, 30.65186413114637531 ) ) ;
#18393=AXIS2_PLACEMENT_3D ( 'NONE', #22109, #12638, #19948 ) ;
#18403=ORIENTED_EDGE ( 'NONE', *, *, #6269, .F. ) ;
#18409=DIRECTION ( 'NONE',  ( 1.000000000000000000, -0.000000000000000000, 6.982962677686266711E-15 ) ) ;
#18435=ORIENTED_EDGE ( 'NONE', *, *, #6533, .F. ) ;
#18437=CARTESIAN_POINT ( 'NONE',  ( -136.3944205523261815, -1073.631384736298514, 32.17229779615536955 ) ) ;
#18469=CIRCLE ( 'NONE', #6917, 2.055000000000001492 ) ;
#18475=CARTESIAN_POINT ( 'NONE',  ( -128.7717867965307903, 86.27213916325827370, -27.99555145635496700 ) ) ;
#18492=CARTESIAN_POINT ( 'NONE',  ( -136.1034519145107993, -1074.167893320492567, -27.57920702976961280 ) ) ;
#18496=ORIENTED_EDGE ( 'NONE', *, *, #2348, .T. ) ;
#18510=CARTESIAN_POINT ( 'NONE',  ( -129.2447185937761844, 85.56171376302357601, 30.81384172145500955 ) ) ;
#18513=AXIS2_PLACEMENT_3D ( 'NONE', #4014, #13255, #22131 ) ;
#18516=CARTESIAN_POINT ( 'NONE',  ( 126.3653543294818178, 77.28387428943173632, -32.05499999999356930 ) ) ;
#18532=CARTESIAN_POINT ( 'NONE',  ( 145.9999999999998010, -209.9999999999996874, 30.00000000000641620 ) ) ;
#18537=CARTESIAN_POINT ( 'NONE',  ( 122.9560050114703387, -1094.375960373424505, -29.67081494451410961 ) ) ;
#18539=DIRECTION ( 'NONE',  ( -1.000000000000000000, 1.408839003528726857E-14, 6.982962677686266711E-15 ) ) ;
#18544=FACE_OUTER_BOUND ( 'NONE', #20596, .T. ) ;
#18552=ORIENTED_EDGE ( 'NONE', *, *, #14777, .T. ) ;
#18559=CARTESIAN_POINT ( 'NONE',  ( 155.0000000000000284, -500.0000000000000000, 30.00000000000001421 ) ) ;
#18560=ADVANCED_FACE ( 'NONE', ( #15914 ), #8195, .F. ) ;
#18564=SHAPE_DEFINITION_REPRESENTATION ( #16548, #4684 ) ;
#18568=ORIENTED_EDGE ( 'NONE', *, *, #15244, .F. ) ;
#18569=ORIENTED_EDGE ( 'NONE', *, *, #12166, .F. ) ;
#18573=DIRECTION ( 'NONE',  ( 1.000000000000000000, -1.408839003528726857E-14, -6.982962677686266711E-15 ) ) ;
#18583=CARTESIAN_POINT ( 'NONE',  ( -127.9021285790837510, 87.55595642181940264, -27.49999999999351985 ) ) ;
#18588=CARTESIAN_POINT ( 'NONE',  ( 125.9649699199272277, -1090.320686186013972, -29.83126738556716262 ) ) ;
#18595=VERTEX_POINT ( 'NONE', #11970 ) ;
#18601=CARTESIAN_POINT ( 'NONE',  ( -134.7157571289267821, -1076.659463591458461, 28.74299381080683347 ) ) ;
#18608=CARTESIAN_POINT ( 'NONE',  ( 124.4701338314438317, -1092.369831568442805, 32.50000000000646594 ) ) ;
#18610=DIRECTION ( 'NONE',  ( 1.110223024625155594E-14, 0.000000000000000000, -1.000000000000000000 ) ) ;
#18623=CARTESIAN_POINT ( 'NONE',  ( 131.6943452429971728, 81.74110354019178715, -31.25700618919314522 ) ) ;
#18624=CIRCLE ( 'NONE', #8242, 2.055000000000001492 ) ;
#18633=DIRECTION ( 'NONE',  ( -6.486615240276975916E-15, -2.585650881802458380E-15, 1.000000000000000000 ) ) ;
#18638=CARTESIAN_POINT ( 'NONE',  ( 123.8018707182395985, -1093.263712923000639, -27.75009929603930559 ) ) ;
#18645=EDGE_CURVE ( 'NONE', #13026, #14427, #10363, .T. ) ;
#18667=EDGE_CURVE ( 'NONE', #223, #13899, #18719, .T. ) ;
#18668=CARTESIAN_POINT ( 'NONE',  ( -122.8605704798721803, 82.74225173005937961, -27.94499999999355921 ) ) ;
#18676=AXIS2_PLACEMENT_3D ( 'NONE', #14452, #10853, #9006 ) ;
#18680=CARTESIAN_POINT ( 'NONE',  ( 119.6158142514527327, -1087.367367941136308, 30.00000000000641620 ) ) ;
#18684=CARTESIAN_POINT ( 'NONE',  ( 145.0000000000000284, 0.000000000000000000, 90.00000000000000000 ) ) ;
#18713=DIRECTION ( 'NONE',  ( 1.350636282998972974E-14, 0.000000000000000000, -1.000000000000000000 ) ) ;
#18717=CARTESIAN_POINT ( 'NONE',  ( -134.8072682999800520, -1076.498424757946395, 28.47118012353581662 ) ) ;
#18719=CIRCLE ( 'NONE', #16050, 145.0000000000000284 ) ;
#18720=DIRECTION ( 'NONE',  ( -1.350636282998972974E-14, 0.000000000000000000, -1.000000000000000000 ) ) ;
#18730=DIRECTION ( 'NONE',  ( -1.000000000000000000, 0.000000000000000000, 0.000000000000000000 ) ) ;
#18732=ORIENTED_EDGE ( 'NONE', *, *, #415, .F. ) ;
#18750=DIRECTION ( 'NONE',  ( 0.9289202219288174023, 0.3702799228849933955, 6.982962677686265922E-15 ) ) ;
#18768=EDGE_LOOP ( 'NONE', ( #14929, #349, #21053, #7577 ) ) ;
#18771=VECTOR ( 'NONE', #14865, 1000.000000000000000 ) ;
#18772=CARTESIAN_POINT ( 'NONE',  ( -129.6400180686271142, -1072.557589128678273, -29.99999999999356248 ) ) ;
#18779=EDGE_CURVE ( 'NONE', #9157, #15889, #22569, .T. ) ;
#18792=DIRECTION ( 'NONE',  ( 1.110223024625155594E-14, 0.000000000000000000, -1.000000000000000000 ) ) ;
#18811=ORIENTED_EDGE ( 'NONE', *, *, #15050, .F. ) ;
#18819=AXIS2_PLACEMENT_3D ( 'NONE', #15071, #20955, #20581 ) ;
#18824=DIRECTION ( 'NONE',  ( 0.000000000000000000, 0.000000000000000000, -1.000000000000000000 ) ) ;
#18827=VERTEX_POINT ( 'NONE', #21910 ) ;
#18833=CARTESIAN_POINT ( 'NONE',  ( 145.0000000000000284, 0.000000000000000000, -90.00000000000000000 ) ) ;
#18838=AXIS2_PLACEMENT_3D ( 'NONE', #14443, #12788, #16355 ) ;
#18840=VECTOR ( 'NONE', #12189, 1000.000000000000114 ) ;
#18847=FACE_OUTER_BOUND ( 'NONE', #19196, .T. ) ;
#18862=CIRCLE ( 'NONE', #10423, 2.499999999999998668 ) ;
#18875=ORIENTED_EDGE ( 'NONE', *, *, #8374, .T. ) ;
#18881=AXIS2_PLACEMENT_3D ( 'NONE', #12409, #3161, #7034 ) ;
#18885=ADVANCED_FACE ( 'NONE', ( #11326 ), #8333, .F. ) ;
#18892=VERTEX_POINT ( 'NONE', #9374 ) ;
#18901=ADVANCED_FACE ( 'NONE', ( #20462 ), #7909, .F. ) ;
#18906=CARTESIAN_POINT ( 'NONE',  ( 194.7499999999997442, -209.9999999999996874, 30.00000000000675726 ) ) ;
#18916=DIRECTION ( 'NONE',  ( 0.6568457881071740889, 0.2618274444092085762, -0.7071067811865532349 ) ) ;
#18927=FACE_OUTER_BOUND ( 'NONE', #15348, .T. ) ;
#18942=CYLINDRICAL_SURFACE ( 'NONE', #12979, 2.500000000000002220 ) ;
#18953=ORIENTED_EDGE ( 'NONE', *, *, #21208, .T. ) ;
#18958=CARTESIAN_POINT ( 'NONE',  ( -136.9913212208051903, -1072.514673757700621, -29.83733181946746882 ) ) ;
#18962=CARTESIAN_POINT ( 'NONE',  ( -134.8618744214600440, -1076.402150461713063, 31.66065886938995533 ) ) ;
#18968=DIRECTION ( 'NONE',  ( -1.110223024625155594E-14, 0.000000000000000000, -1.000000000000000000 ) ) ;
#18978=ORIENTED_EDGE ( 'NONE', *, *, #790, .F. ) ;
#18981=ORIENTED_EDGE ( 'NONE', *, *, #14597, .T. ) ;
#18985=CARTESIAN_POINT ( 'NONE',  ( 131.5594662024485899, 81.95796442703947093, -29.34624901867147884 ) ) ;
#18986=ADVANCED_FACE ( 'NONE', ( #17088, #7789, #22505, #5974, #22625, #13381, #20693 ), #19472, .F. ) ;
#18991=VECTOR ( 'NONE', #5190, 1000.000000000000114 ) ;
#18993=DIRECTION ( 'NONE',  ( -0.9423651898111408132, -0.3345860861306287348, 6.982962677686266711E-15 ) ) ;
#18994=CARTESIAN_POINT ( 'NONE',  ( 124.2727838502227797, -1092.635313011623111, 32.48389983298808659 ) ) ;
#19004=DIRECTION ( 'NONE',  ( -0.000000000000000000, -0.000000000000000000, -1.000000000000000000 ) ) ;
#19015=FACE_OUTER_BOUND ( 'NONE', #21637, .T. ) ;
#19019=CARTESIAN_POINT ( 'NONE',  ( 146.0000000000002558, -210.0000000000003411, -32.05499999999356930 ) ) ;
#19024=AXIS2_PLACEMENT_3D ( 'NONE', #11224, #5750, #3675 ) ;
#19039=DIRECTION ( 'NONE',  ( -1.000000000000000000, 1.408839003528726857E-14, 6.982962677686266711E-15 ) ) ;
#19043=CONICAL_SURFACE ( 'NONE', #7113, 2.055000000000001492, 0.7853981633974633780 ) ;
#19051=CARTESIAN_POINT ( 'NONE',  ( -126.9531799701279766, 88.92639545932793510, 28.11170275877340075 ) ) ;
#19053=EDGE_CURVE ( 'NONE', #19892, #11790, #18862, .T. ) ;
#19064=DIRECTION ( 'NONE',  ( 0.6964005597823107463, -0.7176533009294140397, 6.982962677686265922E-15 ) ) ;
#19107=VECTOR ( 'NONE', #6967, 1000.000000000000114 ) ;
#19109=B_SPLINE_CURVE_WITH_KNOTS ( 'NONE', 3,
 ( #16961, #16833, #290, #426, #14919, #13143, #20561, #16719, #9841, #7646, #22384, #20816, #18985, #17198, #14800, #173, #7527, #20450, #18623, #11915, #2913, #8018, #2568, #10312, #15397, #17656, #17539, #4867 ),
 .UNSPECIFIED., .F., .F.,
 ( 4, 2, 2, 2, 2, 2, 2, 2, 2, 2, 2, 2, 2, 4 ),
 ( 0.007862850516742132811, 0.008354729399060706330, 0.008846608281379278113, 0.009830366046016423415, 0.01032224492833497959, 0.01081412381065353749, 0.01130600269297209540, 0.01179788157529065157, 0.01278163933992775350, 0.01327351822224632702, 0.01376539710456489880, 0.01425727598688347059, 0.01474915486920204237, 0.01573291263383914604 ),
 .UNSPECIFIED. ) ;
#19111=CIRCLE ( 'NONE', #14897, 2.500000000000002220 ) ;
#19112=FACE_OUTER_BOUND ( 'NONE', #7085, .T. ) ;
#19116=DIRECTION ( 'NONE',  ( 0.000000000000000000, 0.000000000000000000, 1.000000000000000000 ) ) ;
#19117=LINE ( 'NONE', #22621, #380 ) ;
#19120=DIRECTION ( 'NONE',  ( -1.000000000000000000, 1.408839003528726857E-14, 6.982962677686266711E-15 ) ) ;
#19125=CIRCLE ( 'NONE', #22588, 2.500000000000002220 ) ;
#19138=CARTESIAN_POINT ( 'NONE',  ( 126.7787238282394924, 77.44864885511604768, 30.00000000000641975 ) ) ;
#19139=ORIENTED_EDGE ( 'NONE', *, *, #19483, .T. ) ;
#19140=ORIENTED_EDGE ( 'NONE', *, *, #4437, .T. ) ;
#19145=CARTESIAN_POINT ( 'NONE',  ( 131.6538433078035268, 81.80629369879993362, 31.11671059283535712 ) ) ;
#19158=DIRECTION ( 'NONE',  ( -0.6964005597823108573, 0.7176533009294141507, -6.982962677686267499E-15 ) ) ;
#19160=EDGE_CURVE ( 'NONE', #6579, #11264, #22388, .T. ) ;
#19162=EDGE_CURVE ( 'NONE', #21974, #22922, #12968, .T. ) ;
#19166=ORIENTED_EDGE ( 'NONE', *, *, #23653, .F. ) ;
#19196=EDGE_LOOP ( 'NONE', ( #11463, #16843, #20147, #4022 ) ) ;
#19198=EDGE_CURVE ( 'NONE', #10799, #13026, #9254, .T. ) ;
#19213=CARTESIAN_POINT ( 'NONE',  ( -123.1824219776882785, 83.04955713735502343, 30.00000000000641975 ) ) ;
#19226=CARTESIAN_POINT ( 'NONE',  ( -146.0000000000000568, -784.4690652294805204, 32.05500000000641592 ) ) ;
#19238=CARTESIAN_POINT ( 'NONE',  ( 123.1512869713297960, -1094.121033843497116, 31.25900233431386965 ) ) ;
#19239=VERTEX_POINT ( 'NONE', #17152 ) ;
#19250=ORIENTED_EDGE ( 'NONE', *, *, #13600, .F. ) ;
#19262=ORIENTED_EDGE ( 'NONE', *, *, #18667, .T. ) ;
#19265=CYLINDRICAL_SURFACE ( 'NONE', #15753, 2.500000000000002220 ) ;
#19271=CARTESIAN_POINT ( 'NONE',  ( -194.7500000000004832, -204.4690652294793836, -29.99999999999322498 ) ) ;
#19272=CIRCLE ( 'NONE', #3069, 2.500000000000002220 ) ;
#19279=LINE ( 'NONE', #15680, #15067 ) ;
#19320=ORIENTED_EDGE ( 'NONE', *, *, #6019, .T. ) ;
#19323=LINE ( 'NONE', #4964, #6741 ) ;
#19326=EDGE_CURVE ( 'NONE', #9785, #1715, #17038, .T. ) ;
#19334=EDGE_CURVE ( 'NONE', #2037, #14427, #4079, .T. ) ;
#19341=VERTEX_POINT ( 'NONE', #17759 ) ;
#19348=EDGE_CURVE ( 'NONE', #14422, #19892, #15947, .T. ) ;
#19349=ORIENTED_EDGE ( 'NONE', *, *, #3708, .T. ) ;
#19373=DIRECTION ( 'NONE',  ( -1.350636282998972974E-14, 0.000000000000000000, -1.000000000000000000 ) ) ;
#19375=AXIS2_PLACEMENT_3D ( 'NONE', #7007, #1, #9174 ) ;
#19380=CARTESIAN_POINT ( 'NONE',  ( 131.9719027401098401, 81.29225469460354248, 28.11255663403418126 ) ) ;
#19381=FACE_OUTER_BOUND ( 'NONE', #23578, .T. ) ;
#19385=DIRECTION ( 'NONE',  ( 0.000000000000000000, 0.000000000000000000, -1.000000000000000000 ) ) ;
#19388=ORIENTED_EDGE ( 'NONE', *, *, #12252, .T. ) ;
#19392=FACE_OUTER_BOUND ( 'NONE', #10623, .T. ) ;
#19396=ORIENTED_EDGE ( 'NONE', *, *, #19963, .T. ) ;
#19406=CARTESIAN_POINT ( 'NONE',  ( -127.7150463208625553, 87.82877071840113103, 32.48389983298811501 ) ) ;
#19408=CARTESIAN_POINT ( 'NONE',  ( -135.1739945062392394, -1075.849084086415360, -27.81095155082704196 ) ) ;
#19411=EDGE_CURVE ( 'NONE', #17109, #6763, #3465, .T. ) ;
#19416=CARTESIAN_POINT ( 'NONE',  ( 134.0852850658434079, 77.75691219176877667, -29.34813586885359271 ) ) ;
#19418=EDGE_CURVE ( 'NONE', #21068, #16414, #7305, .T. ) ;
#19437=DIRECTION ( 'NONE',  ( 0.6964005597823107463, -0.7176533009294141507, 6.982962677686266711E-15 ) ) ;
#19440=CARTESIAN_POINT ( 'NONE',  ( 171.6502151485116485, 95.33502053007514121, -29.99999999999322498 ) ) ;
#19446=FACE_OUTER_BOUND ( 'NONE', #984, .T. ) ;
#19454=PLANE ( 'NONE',  #21978 ) ;
#19464=VERTEX_POINT ( 'NONE', #21954 ) ;
#19471=ORIENTED_EDGE ( 'NONE', *, *, #15096, .F. ) ;
#19472=PLANE ( 'NONE',  #8473 ) ;
#19478=CARTESIAN_POINT ( 'NONE',  ( -129.6400180686271142, -1072.557589128678273, -29.99999999999356248 ) ) ;
#19482=CARTESIAN_POINT ( 'NONE',  ( -146.0000000000000853, -494.4690652294807478, 30.00000000000641620 ) ) ;
#19483=EDGE_CURVE ( 'NONE', #15690, #885, #22690, .T. ) ;
#19493=ORIENTED_EDGE ( 'NONE', *, *, #16399, .F. ) ;
#19499=LINE ( 'NONE', #8187, #5973 ) ;
#19501=CONICAL_SURFACE ( 'NONE', #16068, 2.055000000000001492, 0.7853981633974633780 ) ;
#19502=CARTESIAN_POINT ( 'NONE',  ( 132.1836189744865919, 80.94757571328977974, 27.82811892742372351 ) ) ;
#19508=DIRECTION ( 'NONE',  ( 0.7071067811865320296, 8.659560562355062281E-17, 0.7071067811865631159 ) ) ;
#19509=ORIENTED_EDGE ( 'NONE', *, *, #6318, .F. ) ;
#19512=LINE ( 'NONE', #2964, #6960 ) ;
#19523=DIRECTION ( 'NONE',  ( -0.000000000000000000, -0.000000000000000000, -1.000000000000000000 ) ) ;
#19532=VECTOR ( 'NONE', #17993, 1000.000000000000000 ) ;
#19534=CIRCLE ( 'NONE', #18377, 2.055000000000001492 ) ;
#19539=CARTESIAN_POINT ( 'NONE',  ( 133.9966253006742534, 77.90961723643309256, -31.11320915316591496 ) ) ;
#19545=LINE ( 'NONE', #3004, #5292 ) ;
#19554=CARTESIAN_POINT ( 'NONE',  ( -155.0000000000000284, -494.4690652294799520, -29.99999999999350564 ) ) ;
#19557=LINE ( 'NONE', #20137, #667 ) ;
#19578=ADVANCED_FACE ( 'NONE', ( #11848 ), #16879, .F. ) ;
#19579=DIRECTION ( 'NONE',  ( 0.000000000000000000, 0.000000000000000000, -1.000000000000000000 ) ) ;
#19585=CIRCLE ( 'NONE', #15380, 2.499999999999998668 ) ;
#19595=ORIENTED_EDGE ( 'NONE', *, *, #13701, .T. ) ;
#19599=DIRECTION ( 'NONE',  ( -0.7071067811865416886, 9.961996129952529179E-15, -0.7071067811865532349 ) ) ;
#19603=AXIS2_PLACEMENT_3D ( 'NONE', #4887, #3180, #6458 ) ;
#19604=DIRECTION ( 'NONE',  ( -0.6663528160695909586, -0.2365880903936287138, 0.7071067811865631159 ) ) ;
#19607=CARTESIAN_POINT ( 'NONE',  ( -122.8605704798723082, 82.74225173005861222, 30.00000000000641620 ) ) ;
#19622=CARTESIAN_POINT ( 'NONE',  ( 131.5154891841469862, 82.02850787876555216, 29.67150201188731629 ) ) ;
#19624=CARTESIAN_POINT ( 'NONE',  ( 145.0000000000000284, -500.0000000000000000, -29.99999999999997158 ) ) ;
#19630=DIRECTION ( 'NONE',  ( 1.000000000000000000, -0.000000000000000000, 6.982962677686266711E-15 ) ) ;
#19645=ORIENTED_EDGE ( 'NONE', *, *, #23057, .T. ) ;
#19646=VERTEX_POINT ( 'NONE', #18668 ) ;
#19651=COLOUR_RGB ( '',0.8941176470588234615, 0.8941176470588234615, 0.8941176470588234615 ) ;
#19657=CARTESIAN_POINT ( 'NONE',  ( -146.0000000000001137, -494.4690652294807478, 27.94500000000641649 ) ) ;
#19665=PRODUCT_DEFINITION_FORMATION_WITH_SPECIFIED_SOURCE ( 'ANY', '', #3604, .NOT_KNOWN. ) ;
#19672=CARTESIAN_POINT ( 'NONE',  ( 133.8630869304077748, 78.13886732029796178, -31.53250949154611504 ) ) ;
#19685=ORIENTED_EDGE ( 'NONE', *, *, #2690, .F. ) ;
#19691=EDGE_LOOP ( 'NONE', ( #6311, #1556, #19140, #13656 ) ) ;
#19693=VERTEX_POINT ( 'NONE', #23148 ) ;
#19707=ORIENTED_EDGE ( 'NONE', *, *, #13098, .F. ) ;
#19733=DIRECTION ( 'NONE',  ( 1.000000000000000000, -0.000000000000000000, 6.982962677686266711E-15 ) ) ;
#19734=ORIENTED_EDGE ( 'NONE', *, *, #16570, .T. ) ;
#19740=ORIENTED_EDGE ( 'NONE', *, *, #2690, .T. ) ;
#19748=CARTESIAN_POINT ( 'NONE',  ( -146.0000000000005116, -494.4690652294800657, -29.99999999999356604 ) ) ;
#19751=CARTESIAN_POINT ( 'NONE',  ( -123.1824219776881648, 83.04955713735580503, -29.99999999999356248 ) ) ;
#19752=LINE ( 'NONE', #19986, #20590 ) ;
#19756=ADVANCED_FACE ( 'NONE', ( #23511 ), #4557, .F. ) ;
#19761=DIRECTION ( 'NONE',  ( 0.9289202219288174023, 0.3702799228849934510, 6.982962677686266711E-15 ) ) ;
#19765=ORIENTED_EDGE ( 'NONE', *, *, #19836, .T. ) ;
#19767=CARTESIAN_POINT ( 'NONE',  ( -155.0000000000000284, -784.4690652294798383, -29.99999999999350564 ) ) ;
#19775=EDGE_CURVE ( 'NONE', #2188, #6623, #2243, .T. ) ;
#19778=CARTESIAN_POINT ( 'NONE',  ( -134.5810953439730326, -1076.895678479287426, -30.65604281379823703 ) ) ;
#19781=MANIFOLD_SOLID_BREP ( 'Cavity1', #1735 ) ;
#19784=CARTESIAN_POINT ( 'NONE',  ( -194.7500000000004832, -784.4690652294792699, -29.99999999999322498 ) ) ;
#19787=CARTESIAN_POINT ( 'NONE',  ( 133.6912351773694354, 78.43256762916455216, -28.11073331261974317 ) ) ;
#19795=EDGE_CURVE ( 'NONE', #5229, #8689, #8422, .T. ) ;
#19799=CONICAL_SURFACE ( 'NONE', #9398, 2.055000000000001492, 0.7853981633974633780 ) ;
#19803=DIRECTION ( 'NONE',  ( 1.000000000000000000, 0.000000000000000000, 0.000000000000000000 ) ) ;
#19825=VECTOR ( 'NONE', #12537, 1000.000000000000114 ) ;
#19828=CARTESIAN_POINT ( 'NONE',  ( -122.8605704798723082, 82.74225173005861222, 30.00000000000641620 ) ) ;
#19836=EDGE_CURVE ( 'NONE', #223, #9869, #6101, .T. ) ;
#19837=ORIENTED_EDGE ( 'NONE', *, *, #18779, .T. ) ;
#19844=DIRECTION ( 'NONE',  ( 0.6964005597823107463, -0.7176533009294140397, 6.982962677686265922E-15 ) ) ;
#19849=CARTESIAN_POINT ( 'NONE',  ( 133.6256533058501077, 78.54427823740881820, 28.00660068667233560 ) ) ;
#19862=DIRECTION ( 'NONE',  ( -0.7071067811865416886, 9.961996129952529179E-15, -0.7071067811865532349 ) ) ;
#19867=DIRECTION ( 'NONE',  ( -0.7232617928448825673, 0.6905739489807055653, 6.982962677686265922E-15 ) ) ;
#19870=DIRECTION ( 'NONE',  ( 1.000000000000000000, -0.000000000000000000, 6.982962677686266711E-15 ) ) ;
#19874=CIRCLE ( 'NONE', #20617, 2.499999999999998668 ) ;
#19883=CIRCLE ( 'NONE', #5558, 2.499999999999998668 ) ;
#19886=DIRECTION ( 'NONE',  ( 0.9289202219288174023, 0.3702799228849934510, 6.982962677686266711E-15 ) ) ;
#19889=CARTESIAN_POINT ( 'NONE',  ( -194.7500000000000284, -494.4690652294800657, 30.00000000000675726 ) ) ;
#19892=VERTEX_POINT ( 'NONE', #17217 ) ;
#19900=ORIENTED_EDGE ( 'NONE', *, *, #21375, .T. ) ;
#19907=DIRECTION ( 'NONE',  ( -0.6663528160696001734, -0.2365880903936319335, -0.7071067811865532349 ) ) ;
#19910=CARTESIAN_POINT ( 'NONE',  ( -126.4560199014025414, 89.63188623867986848, -29.83733181946746527 ) ) ;
#19917=DIRECTION ( 'NONE',  ( -0.6663528160696001734, -0.2365880903936319335, -0.7071067811865532349 ) ) ;
#19919=CARTESIAN_POINT ( 'NONE',  ( -146.4450000000000784, -494.4690652294807478, 30.00000000000641975 ) ) ;
#19928=VERTEX_POINT ( 'NONE', #15425 ) ;
#19937=FACE_OUTER_BOUND ( 'NONE', #17597, .T. ) ;
#19938=AXIS2_PLACEMENT_3D ( 'NONE', #9909, #12110, #1060 ) ;
#19948=DIRECTION ( 'NONE',  ( 5.050510105632271307E-15, -4.822252111914687128E-15, 1.000000000000000000 ) ) ;
#19960=CARTESIAN_POINT ( 'NONE',  ( 133.6917068022185617, 78.43176171823573384, 28.11170275877340785 ) ) ;
#19963=EDGE_CURVE ( 'NONE', #11453, #21308, #20389, .T. ) ;
#19975=CARTESIAN_POINT ( 'NONE',  ( 155.0000000000000284, -209.9999999999996874, 30.00000000000648015 ) ) ;
#19979=DIRECTION ( 'NONE',  ( -6.753181414994864868E-15, 6.753181414994864868E-15, -1.000000000000000000 ) ) ;
#19981=DIRECTION ( 'NONE',  ( -1.000000000000000000, -2.775557561562891351E-17, 0.000000000000000000 ) ) ;
#19986=CARTESIAN_POINT ( 'NONE',  ( 155.0000000000000284, -500.0000000000000000, -27.49999999999996803 ) ) ;
#19987=CIRCLE ( 'NONE', #21151, 2.055000000000001492 ) ;
#19988=ORIENTED_EDGE ( 'NONE', *, *, #16570, .F. ) ;
#20000=DIRECTION ( 'NONE',  ( 1.110223024625155594E-14, 0.000000000000000000, -1.000000000000000000 ) ) ;
#20023=VERTEX_POINT ( 'NONE', #14207 ) ;
#20029=VECTOR ( 'NONE', #19844, 1000.000000000000114 ) ;
#20030=AXIS2_PLACEMENT_3D ( 'NONE', #5328, #22343, #3869 ) ;
#20036=AXIS2_PLACEMENT_3D ( 'NONE', #14458, #19981, #8655 ) ;
#20042=DIRECTION ( 'NONE',  ( -1.000000000000000000, 1.408839003528726857E-14, 6.982962677686266711E-15 ) ) ;
#20051=AXIS2_PLACEMENT_3D ( 'NONE', #18772, #6114, #11707 ) ;
#20060=CARTESIAN_POINT ( 'NONE',  ( -123.1824219776881648, 83.04955713735579081, -27.49999999999356248 ) ) ;
#20066=VECTOR ( 'NONE', #11730, 1000.000000000000000 ) ;
#20072=CARTESIAN_POINT ( 'NONE',  ( 146.0000000000001990, -801.0618695410406644, -27.94499999999356632 ) ) ;
#20085=EDGE_LOOP ( 'NONE', ( #23391, #13289, #16386, #9629 ) ) ;
#20089=CARTESIAN_POINT ( 'NONE',  ( 133.0106877214035137, 79.58129789419636779, 32.48389983298810790 ) ) ;
#20093=CARTESIAN_POINT ( 'NONE',  ( 155.0000000000000568, -801.0618695410406644, -27.49999999999350209 ) ) ;
#20099=ORIENTED_EDGE ( 'NONE', *, *, #6670, .T. ) ;
#20110=CARTESIAN_POINT ( 'NONE',  ( 0.000000000000000000, 0.000000000000000000, 90.00000000000000000 ) ) ;
#20118=LINE ( 'NONE', #6981, #20165 ) ;
#20119=VERTEX_POINT ( 'NONE', #3764 ) ;
#20126=DIRECTION ( 'NONE',  ( -1.000000000000000000, 1.408839003528726857E-14, 6.982962677686266711E-15 ) ) ;
#20131=EDGE_CURVE ( 'NONE', #13840, #23140, #9296, .T. ) ;
#20136=DIRECTION ( 'NONE',  ( -1.000000000000000000, 1.408839003528726857E-14, 6.982962677686266711E-15 ) ) ;
#20137=CARTESIAN_POINT ( 'NONE',  ( -158.1195828810603246, 116.4077317428680090, 27.50000000000675371 ) ) ;
#20147=ORIENTED_EDGE ( 'NONE', *, *, #16202, .T. ) ;
#20164=DIRECTION ( 'NONE',  ( -0.7232617928448825673, 0.6905739489807055653, 6.982962677686266711E-15 ) ) ;
#20165=VECTOR ( 'NONE', #12918, 999.9999999999998863 ) ;
#20171=EDGE_LOOP ( 'NONE', ( #20292, #12919, #15439, #7040 ) ) ;
#20179=ORIENTED_EDGE ( 'NONE', *, *, #20310, .F. ) ;
#20195=CIRCLE ( 'NONE', #10589, 2.055000000000001492 ) ;
#20224=FACE_OUTER_BOUND ( 'NONE', #6710, .T. ) ;
#20227=CARTESIAN_POINT ( 'NONE',  ( -145.0000000000000284, -1000.000000000000000, 90.00000000000000000 ) ) ;
#20250=CARTESIAN_POINT ( 'NONE',  ( -136.3934655611483322, -1073.633154336009738, 27.82653936295263719 ) ) ;
#20257=DIRECTION ( 'NONE',  ( -1.110223024625155594E-14, 0.000000000000000000, -1.000000000000000000 ) ) ;
#20280=CARTESIAN_POINT ( 'NONE',  ( 125.2206635291104249, -1091.349901830162707, -32.17188107257626939 ) ) ;
#20287=ORIENTED_EDGE ( 'NONE', *, *, #8188, .F. ) ;
#20292=ORIENTED_EDGE ( 'NONE', *, *, #16200, .F. ) ;
#20299=ORIENTED_EDGE ( 'NONE', *, *, #19162, .T. ) ;
#20300=CARTESIAN_POINT ( 'NONE',  ( 124.5680376182010320, -1092.237904323006205, 32.50000000000647304 ) ) ;
#20310=EDGE_CURVE ( 'NONE', #590, #23044, #13130, .T. ) ;
#20318=DIRECTION ( 'NONE',  ( -1.000000000000000000, -2.775557561562891351E-17, 0.000000000000000000 ) ) ;
#20319=DIRECTION ( 'NONE',  ( 1.000000000000000000, -0.000000000000000000, -0.000000000000000000 ) ) ;
#20322=AXIS2_PLACEMENT_3D ( 'NONE', #10681, #11035, #7028 ) ;
#20324=DIRECTION ( 'NONE',  ( 0.9289202219288174023, 0.3702799228849934510, 6.982962677686266711E-15 ) ) ;
#20328=VERTEX_POINT ( 'NONE', #6306 ) ;
#20331=CARTESIAN_POINT ( 'NONE',  ( -175.1609685624542294, -1088.719770019218458, -27.49999999999322498 ) ) ;
#20334=CARTESIAN_POINT ( 'NONE',  ( 123.3268328482423044, -1093.890927824661958, -28.34359615383078790 ) ) ;
#20345=DIRECTION ( 'NONE',  ( 1.110223024625155594E-14, 0.000000000000000000, -1.000000000000000000 ) ) ;
#20356=VECTOR ( 'NONE', #18916, 1000.000000000000114 ) ;
#20358=CARTESIAN_POINT ( 'NONE',  ( 126.3653543294818178, 77.28387428943173632, -29.99999999999356604 ) ) ;
#20359=AXIS2_PLACEMENT_3D ( 'NONE', #20800, #8334, #18730 ) ;
#20361=EDGE_CURVE ( 'NONE', #19693, #14422, #4551, .T. ) ;
#20372=DIRECTION ( 'NONE',  ( -1.000000000000000000, 1.408839003528726857E-14, 6.982962677686266711E-15 ) ) ;
#20380=VECTOR ( 'NONE', #9774, 1000.000000000000000 ) ;
#20389=CIRCLE ( 'NONE', #13512, 2.499999999999998668 ) ;
#20396=DIRECTION ( 'NONE',  ( 0.000000000000000000, 0.000000000000000000, -1.000000000000000000 ) ) ;
#20408=ORIENTED_EDGE ( 'NONE', *, *, #4437, .F. ) ;
#20412=B_SPLINE_CURVE_WITH_KNOTS ( 'NONE', 3,
 ( #21950, #1774, #221, #22064, #5531, #3018, #20250, #9164, #22178, #2012, #10434, #3700, #17779, #11117, #2732, #5422, #1223, #9402, #8594, #5295, #7575, #15966, #16523, #11001, #12833, #18437, #23310, #3481, #6778, #21501, #10891, #9047 ),
 .UNSPECIFIED., .F., .F.,
 ( 4, 2, 2, 2, 2, 2, 2, 2, 2, 2, 2, 2, 2, 2, 2, 4 ),
 ( 2.964296775167216948E-17, 0.0004914281572964689527, 0.0009828563145929084151, 0.001474284471889347877, 0.001965712629185786906, 0.002457140786482226585, 0.002948568943778665831, 0.003931425258371301461, 0.004422853415667624480, 0.004914281572963947499, 0.005405709730260270518, 0.005897137887556594404, 0.006388566044852917424, 0.006879994202149240443, 0.007371422359445564329, 0.007862850516741886481 ),
 .UNSPECIFIED. ) ;
#20418=CARTESIAN_POINT ( 'NONE',  ( -136.8702482660837347, -1072.742966597997338, -31.11320915316586522 ) ) ;
#20424=ORIENTED_EDGE ( 'NONE', *, *, #12364, .T. ) ;
#20430=DIRECTION ( 'NONE',  ( 1.350636282998972974E-14, 0.000000000000000000, -1.000000000000000000 ) ) ;
#20434=ADVANCED_FACE ( 'NONE', ( #21641 ), #7247, .F. ) ;
#20438=CARTESIAN_POINT ( 'NONE',  ( -128.9672686250725633, 85.97940096925731268, 31.66065886938990914 ) ) ;
#20450=CARTESIAN_POINT ( 'NONE',  ( 131.6528213848855273, 81.80793830425525925, -31.11299551804357932 ) ) ;
#20453=CARTESIAN_POINT ( 'NONE',  ( 133.9969223633119384, 77.90910650221383094, 31.11216498479350179 ) ) ;
#20456=DIRECTION ( 'NONE',  ( -1.000000000000000000, -2.775557561562891351E-17, 0.000000000000000000 ) ) ;
#20462=FACE_OUTER_BOUND ( 'NONE', #4153, .T. ) ;
#20471=CARTESIAN_POINT ( 'NONE',  ( 145.0000000000000284, -500.0000000000000000, -29.99999999999997158 ) ) ;
#20474=FACE_OUTER_BOUND ( 'NONE', #4500, .T. ) ;
#20478=FACE_OUTER_BOUND ( 'NONE', #21795, .T. ) ;
#20505=DIRECTION ( 'NONE',  ( 6.753181414994864868E-15, 0.000000000000000000, -1.000000000000000000 ) ) ;
#20507=CARTESIAN_POINT ( 'NONE',  ( -127.5331898753161681, 88.09262935741045908, 27.57867027829822959 ) ) ;
#20511=VECTOR ( 'NONE', #250, 1000.000000000000000 ) ;
#20516=CARTESIAN_POINT ( 'NONE',  ( -129.1300454301534444, 85.73470730629067305, -28.73951976925631868 ) ) ;
#20518=ADVANCED_FACE ( 'NONE', ( #9201 ), #12860, .F. ) ;
#20524=CARTESIAN_POINT ( 'NONE',  ( -145.0000000000000284, -1.110223024625156540E-13, 90.00000000000000000 ) ) ;
#20525=ORIENTED_EDGE ( 'NONE', *, *, #17142, .F. ) ;
#20528=DIRECTION ( 'NONE',  ( 0.9289202219288174023, 0.3702799228849934510, 6.982962677686266711E-15 ) ) ;
#20535=EDGE_CURVE ( 'NONE', #4200, #15958, #13848, .T. ) ;
#20537=CARTESIAN_POINT ( 'NONE',  ( -134.6777706902592229, -1076.726150876685551, 31.11671059283538554 ) ) ;
#20542=CARTESIAN_POINT ( 'NONE',  ( 119.6158142514525622, -1087.367367941136990, -29.99999999999356604 ) ) ;
#20544=AXIS2_PLACEMENT_3D ( 'NONE', #4689, #4800, #3107 ) ;
#20548=CARTESIAN_POINT ( 'NONE',  ( -129.1311602790088102, 85.73302760282668089, 28.74299381080684412 ) ) ;
#20561=CARTESIAN_POINT ( 'NONE',  ( 132.0350058597971952, 81.18997658688611807, -27.99555145635497411 ) ) ;
#20566=CARTESIAN_POINT ( 'NONE',  ( -129.2206655591605511, -1072.408698320350595, 30.00000000000641620 ) ) ;
#20567=CARTESIAN_POINT ( 'NONE',  ( 123.5476367174099011, -1093.600214943837045, 31.99235058689527733 ) ) ;
#20580=CARTESIAN_POINT ( 'NONE',  ( -129.2206655591611764, -1072.408698320350140, -32.05499999999358351 ) ) ;
#20581=DIRECTION ( 'NONE',  ( 1.350636282998972974E-14, 0.000000000000000000, -1.000000000000000000 ) ) ;
#20590=VECTOR ( 'NONE', #3201, 1000.000000000000000 ) ;
#20596=EDGE_LOOP ( 'NONE', ( #4556, #18569, #12467, #6950 ) ) ;
#20611=AXIS2_PLACEMENT_3D ( 'NONE', #6419, #19437, #13824 ) ;
#20617=AXIS2_PLACEMENT_3D ( 'NONE', #480, #15220, #7587 ) ;
#20624=FACE_OUTER_BOUND ( 'NONE', #1817, .T. ) ;
#20650=ORIENTED_EDGE ( 'NONE', *, *, #1946, .T. ) ;
#20653=ORIENTED_EDGE ( 'NONE', *, *, #3116, .T. ) ;
#20655=DIRECTION ( 'NONE',  ( -1.000000000000000000, 1.408839003528726857E-14, 6.982962677686266711E-15 ) ) ;
#20687=CARTESIAN_POINT ( 'NONE',  ( 155.0000000000000284, -209.9999999999996874, 27.50000000000647660 ) ) ;
#20693=FACE_OUTER_BOUND ( 'NONE', #18163, .T. ) ;
#20699=DIRECTION ( 'NONE',  ( 1.110223024625157172E-14, 0.000000000000000000, -1.000000000000000000 ) ) ;
#20707=VECTOR ( 'NONE', #4073, 1000.000000000000114 ) ;
#20712=CARTESIAN_POINT ( 'NONE',  ( -122.8605704798723224, 82.74225173005862644, 27.94500000000641649 ) ) ;
#20727=CONICAL_SURFACE ( 'NONE', #10346, 2.055000000000001492, 0.7853981633974633780 ) ;
#20736=DIRECTION ( 'NONE',  ( -1.110223024625155594E-14, 0.000000000000000000, -1.000000000000000000 ) ) ;
#20741=VECTOR ( 'NONE', #11548, 1000.000000000000114 ) ;
#20746=LINE ( 'NONE', #9536, #7480 ) ;
#20774=VERTEX_POINT ( 'NONE', #12333 ) ;
#20775=CARTESIAN_POINT ( 'NONE',  ( -136.3934655611484743, -1073.633154336008602, -32.17346063704741965 ) ) ;
#20789=AXIS2_PLACEMENT_3D ( 'NONE', #14842, #22421, #4055 ) ;
#20800=CARTESIAN_POINT ( 'NONE',  ( 0.000000000000000000, -1000.000000000000000, 90.00000000000000000 ) ) ;
#20808=VECTOR ( 'NONE', #19862, 1000.000000000000114 ) ;
#20816=CARTESIAN_POINT ( 'NONE',  ( 131.5858269427386915, 81.91565353609531996, -29.18615827854495848 ) ) ;
#20821=EDGE_CURVE ( 'NONE', #10033, #8499, #17720, .T. ) ;
#20825=CARTESIAN_POINT ( 'NONE',  ( 123.2641556675340127, -1093.973169342142455, 28.46749050845384943 ) ) ;
#20846=ORIENTED_EDGE ( 'NONE', *, *, #17263, .F. ) ;
#20862=LINE ( 'NONE', #13546, #20356 ) ;
#20873=CARTESIAN_POINT ( 'NONE',  ( -146.0000000000000853, -784.4690652294805204, 30.00000000000641620 ) ) ;
#20876=ORIENTED_EDGE ( 'NONE', *, *, #15584, .T. ) ;
#20882=EDGE_CURVE ( 'NONE', #15114, #23044, #3920, .T. ) ;
#20886=CARTESIAN_POINT ( 'NONE',  ( -126.4560199014029251, 89.63188623867937110, 30.16266818053252052 ) ) ;
#20889=ORIENTED_EDGE ( 'NONE', *, *, #14805, .T. ) ;
#20890=DIRECTION ( 'NONE',  ( -6.753181414994864868E-15, 6.753181414994864868E-15, -1.000000000000000000 ) ) ;
#20894=FACE_OUTER_BOUND ( 'NONE', #6692, .T. ) ;
#20898=ORIENTED_EDGE ( 'NONE', *, *, #4252, .T. ) ;
#20905=ORIENTED_EDGE ( 'NONE', *, *, #6095, .T. ) ;
#20929=EDGE_CURVE ( 'NONE', #20119, #907, #2652, .T. ) ;
#20949=CARTESIAN_POINT ( 'NONE',  ( 146.4449999999997942, -801.0618695410399823, 30.00000000000641975 ) ) ;
#20955=DIRECTION ( 'NONE',  ( 1.000000000000000000, -0.000000000000000000, 6.982962677686266711E-15 ) ) ;
#20968=CIRCLE ( 'NONE', #5539, 145.0000000000000284 ) ;
#20971=CARTESIAN_POINT ( 'NONE',  ( -194.7500000000004547, -494.4690652294794404, -27.49999999999322498 ) ) ;
#20974=DIRECTION ( 'NONE',  ( 1.000000000000000000, -0.000000000000000000, -0.000000000000000000 ) ) ;
#20979=EDGE_CURVE ( 'NONE', #18017, #10087, #21548, .T. ) ;
#20992=EDGE_LOOP ( 'NONE', ( #14915, #2586, #23024, #15701 ) ) ;
#21011=AXIS2_PLACEMENT_3D ( 'NONE', #22715, #4364, #1851 ) ;
#21023=EDGE_LOOP ( 'NONE', ( #9404, #16555, #4772, #12690 ) ) ;
#21053=ORIENTED_EDGE ( 'NONE', *, *, #12405, .T. ) ;
#21057=CARTESIAN_POINT ( 'NONE',  ( 123.0250976530554539, -1094.285891978964173, 30.80845853161007497 ) ) ;
#21068=VERTEX_POINT ( 'NONE', #4528 ) ;
#21075=EDGE_CURVE ( 'NONE', #22831, #18827, #1495, .T. ) ;
#21076=DIRECTION ( 'NONE',  ( -1.350636282998972974E-14, 0.000000000000000000, -1.000000000000000000 ) ) ;
#21080=ADVANCED_FACE ( 'NONE', ( #15183 ), #3017, .F. ) ;
#21087=CYLINDRICAL_SURFACE ( 'NONE', #8297, 2.500000000000002220 ) ;
#21091=ORIENTED_EDGE ( 'NONE', *, *, #14644, .T. ) ;
#21112=AXIS2_PLACEMENT_3D ( 'NONE', #22050, #19886, #20345 ) ;
#21113=ORIENTED_EDGE ( 'NONE', *, *, #21802, .F. ) ;
#21122=AXIS2_PLACEMENT_3D ( 'NONE', #23529, #11654, #732 ) ;
#21144=EDGE_CURVE ( 'NONE', #846, #15958, #3072, .T. ) ;
#21151=AXIS2_PLACEMENT_3D ( 'NONE', #6520, #16820, #11536 ) ;
#21153=AXIS2_PLACEMENT_3D ( 'NONE', #8727, #16091, #12623 ) ;
#21166=AXIS2_PLACEMENT_3D ( 'NONE', #20471, #13036, #11333 ) ;
#21170=CIRCLE ( 'NONE', #17706, 2.499999999999998668 ) ;
#21180=EDGE_CURVE ( 'NONE', #13741, #12953, #16536, .T. ) ;
#21185=DIRECTION ( 'NONE',  ( 0.6964005597823107463, -0.7176533009294140397, 6.982962677686265922E-15 ) ) ;
#21194=CONICAL_SURFACE ( 'NONE', #3041, 2.055000000000001492, 0.7853981633974633780 ) ;
#21196=CONICAL_SURFACE ( 'NONE', #16955, 2.055000000000001492, 0.7853981633974633780 ) ;
#21203=DIRECTION ( 'NONE',  ( 1.000000000000000000, 0.000000000000000000, -0.000000000000000000 ) ) ;
#21207=EDGE_LOOP ( 'NONE', ( #6040, #16108, #13387, #19765 ) ) ;
#21208=EDGE_CURVE ( 'NONE', #19693, #11790, #15898, .T. ) ;
#21217=CIRCLE ( 'NONE', #5805, 2.055000000000001492 ) ;
#21228=ORIENTED_EDGE ( 'NONE', *, *, #1729, .F. ) ;
#21237=AXIS2_PLACEMENT_3D ( 'NONE', #12209, #6729, #14010 ) ;
#21245=ADVANCED_FACE ( 'NONE', ( #14340 ), #12296, .F. ) ;
#21246=FACE_OUTER_BOUND ( 'NONE', #11748, .T. ) ;
#21251=VERTEX_POINT ( 'NONE', #10219 ) ;
#21256=ORIENTED_EDGE ( 'NONE', *, *, #8188, .T. ) ;
#21257=CARTESIAN_POINT ( 'NONE',  ( 132.9250442248338118, 79.72427207779705327, -27.49999999999352340 ) ) ;
#21262=DIRECTION ( 'NONE',  ( 0.000000000000000000, 5.551115123125777969E-15, -1.000000000000000000 ) ) ;
#21276=CARTESIAN_POINT ( 'NONE',  ( -146.4450000000005332, -494.4690652294800657, -29.99999999999356248 ) ) ;
#21280=FACE_OUTER_BOUND ( 'NONE', #10022, .T. ) ;
#21283=DIRECTION ( 'NONE',  ( -0.7232617928448825673, 0.6905739489807055653, 6.982962677686266711E-15 ) ) ;
#21297=CYLINDRICAL_SURFACE ( 'NONE', #11461, 2.500000000000002220 ) ;
#21301=FACE_BOUND ( 'NONE', #4608, .T. ) ;
#21303=ORIENTED_EDGE ( 'NONE', *, *, #14597, .F. ) ;
#21307=DIRECTION ( 'NONE',  ( 0.6964005597823107463, -0.7176533009294141507, 6.982962677686266711E-15 ) ) ;
#21308=VERTEX_POINT ( 'NONE', #12538 ) ;
#21314=EDGE_CURVE ( 'NONE', #4934, #9588, #12735, .T. ) ;
#21323=CIRCLE ( 'NONE', #5508, 2.500000000000002220 ) ;
#21326=DIRECTION ( 'NONE',  ( 0.6568457881071649851, 0.2618274444092050790, 0.7071067811865631159 ) ) ;
#21328=CARTESIAN_POINT ( 'NONE',  ( 132.4204480437711879, 80.55959301515328264, 32.37380477188060723 ) ) ;
#21333=DIRECTION ( 'NONE',  ( -5.551115123125785858E-15, 5.551115123125785858E-15, -1.000000000000000000 ) ) ;
#21339=DIRECTION ( 'NONE',  ( 1.110223024625157172E-14, 0.000000000000000000, -1.000000000000000000 ) ) ;
#21342=DIRECTION ( 'NONE',  ( 2.775557561562891351E-17, -1.000000000000000000, 0.000000000000000000 ) ) ;
#21355=CARTESIAN_POINT ( 'NONE',  ( -126.7581711459448712, 89.20411804604300698, 28.46749050845386009 ) ) ;
#21358=ORIENTED_EDGE ( 'NONE', *, *, #21985, .T. ) ;
#21367=FACE_BOUND ( 'NONE', #5598, .T. ) ;
#21375=EDGE_CURVE ( 'NONE', #11798, #10799, #11061, .T. ) ;
#21383=AXIS2_PLACEMENT_3D ( 'NONE', #16866, #2005, #9393 ) ;
#21393=ORIENTED_EDGE ( 'NONE', *, *, #16315, .T. ) ;
#21396=EDGE_LOOP ( 'NONE', ( #7962, #12667, #16547, #22704 ) ) ;
#21418=DIRECTION ( 'NONE',  ( -1.000000000000000000, -2.775557561562891351E-17, 0.000000000000000000 ) ) ;
#21432=VERTEX_POINT ( 'NONE', #8249 ) ;
#21441=ADVANCED_FACE ( 'NONE', ( #19446 ), #17649, .F. ) ;
#21445=DIRECTION ( 'NONE',  ( 6.982962677686266711E-15, -9.837870180509810443E-29, 1.000000000000000000 ) ) ;
#21447=CARTESIAN_POINT ( 'NONE',  ( 132.8404720734533555, 79.86494211668889420, -27.49999999999351985 ) ) ;
#21452=EDGE_LOOP ( 'NONE', ( #5843, #18132, #1931, #15519 ) ) ;
#21458=FACE_OUTER_BOUND ( 'NONE', #21207, .T. ) ;
#21461=ORIENTED_EDGE ( 'NONE', *, *, #18076, .F. ) ;
#21463=CIRCLE ( 'NONE', #7966, 2.500000000000002220 ) ;
#21478=EDGE_CURVE ( 'NONE', #11453, #20774, #15979, .T. ) ;
#21484=CARTESIAN_POINT ( 'NONE',  ( 133.8109447024532983, 78.22816056888444791, -28.34359615383082343 ) ) ;
#21501=CARTESIAN_POINT ( 'NONE',  ( -135.9487776228373264, -1074.451030117130358, 32.48389983298811501 ) ) ;
#21502=CARTESIAN_POINT ( 'NONE',  ( -146.0000000000005400, -494.4690652294800657, -32.05499999999356930 ) ) ;
#21503=EDGE_CURVE ( 'NONE', #8260, #846, #17701, .T. ) ;
#21504=EDGE_LOOP ( 'NONE', ( #7224, #13604, #12029, #4582 ) ) ;
#21510=CARTESIAN_POINT ( 'NONE',  ( 124.8578076529639702, -1091.845273256946484, -27.57873596473014643 ) ) ;
#21519=DIRECTION ( 'NONE',  ( -0.9423651898111408132, -0.3345860861306287348, 6.982962677686266711E-15 ) ) ;
#21524=ORIENTED_EDGE ( 'NONE', *, *, #7703, .T. ) ;
#21537=CARTESIAN_POINT ( 'NONE',  ( -129.2813770747751789, 85.50638651249015254, -30.65604281379820861 ) ) ;
#21548=CIRCLE ( 'NONE', #5740, 2.055000000000001492 ) ;
#21553=CARTESIAN_POINT ( 'NONE',  ( 145.9999999999998010, -801.0618695410399823, 30.00000000000641620 ) ) ;
#21554=CIRCLE ( 'NONE', #1478, 2.499999999999998668 ) ;
#21565=DIRECTION ( 'NONE',  ( 1.000000000000000000, -1.408839003528726857E-14, -6.982962677686266711E-15 ) ) ;
#21571=DIRECTION ( 'NONE',  ( -1.000000000000000000, 1.408839003528726857E-14, 6.982962677686266711E-15 ) ) ;
#21609=EDGE_LOOP ( 'NONE', ( #13797, #4121, #13050, #22302 ) ) ;
#21610=CARTESIAN_POINT ( 'NONE',  ( -134.6139742523217251, -1076.838024977515715, -29.18615827854494782 ) ) ;
#21618=VERTEX_POINT ( 'NONE', #36 ) ;
#21619=CARTESIAN_POINT ( 'NONE',  ( 132.9260832389180962, 79.72254387117985175, -32.49999999999352696 ) ) ;
#21621=AXIS2_PLACEMENT_3D ( 'NONE', #19138, #6596, #803 ) ;
#21631=EDGE_CURVE ( 'NONE', #14223, #17523, #7383, .T. ) ;
#21637=EDGE_LOOP ( 'NONE', ( #20287, #12286, #2713, #2625 ) ) ;
#21641=FACE_OUTER_BOUND ( 'NONE', #23097, .T. ) ;
#21662=CARTESIAN_POINT ( 'NONE',  ( -128.0900118278588877, 87.28149574061879434, -32.49999999999351985 ) ) ;
#21664=ORIENTED_EDGE ( 'NONE', *, *, #11595, .F. ) ;
#21677=EDGE_CURVE ( 'NONE', #21251, #223, #23570, .T. ) ;
#21679=DIRECTION ( 'NONE',  ( 6.982962677686266711E-15, -9.837870180509810443E-29, 1.000000000000000000 ) ) ;
#21682=EDGE_CURVE ( 'NONE', #5008, #15114, #14199, .T. ) ;
#21683=AXIS2_PLACEMENT_3D ( 'NONE', #20358, #15089, #3826 ) ;
#21695=CARTESIAN_POINT ( 'NONE',  ( -145.0000000000000284, -999.9999999999998863, -90.00000000000000000 ) ) ;
#21698=CARTESIAN_POINT ( 'NONE',  ( 194.7500000000002274, -801.0618695410406644, -32.49999999999322853 ) ) ;
#21702=ORIENTED_EDGE ( 'NONE', *, *, #18259, .T. ) ;
#21714=ORIENTED_EDGE ( 'NONE', *, *, #11972, .T. ) ;
#21715=ADVANCED_FACE ( 'NONE', ( #19937 ), #3614, .F. ) ;
#21729=CARTESIAN_POINT ( 'NONE',  ( -127.5331898753157276, 88.09262935741099909, -32.42132972170175265 ) ) ;
#21750=DIRECTION ( 'NONE',  ( 0.000000000000000000, 0.000000000000000000, -1.000000000000000000 ) ) ;
#21755=VECTOR ( 'NONE', #104, 1000.000000000000114 ) ;
#21757=ORIENTED_EDGE ( 'NONE', *, *, #17276, .F. ) ;
#21760=CARTESIAN_POINT ( 'NONE',  ( 119.9257125005558606, -1087.686723660049893, 32.50000000000641620 ) ) ;
#21793=DIRECTION ( 'NONE',  ( 1.000000000000000000, 0.000000000000000000, 0.000000000000000000 ) ) ;
#21795=EDGE_LOOP ( 'NONE', ( #17774, #22548, #18217, #14296 ) ) ;
#21802=EDGE_CURVE ( 'NONE', #10087, #20023, #13332, .T. ) ;
#21804=( NAMED_UNIT ( * ) PLANE_ANGLE_UNIT ( ) SI_UNIT ( $, .RADIAN. ) );
#21805=DIRECTION ( 'NONE',  ( 1.000000000000000000, -0.000000000000000000, -0.000000000000000000 ) ) ;
#21806=CARTESIAN_POINT ( 'NONE',  ( 155.0000000000000284, 2.775557561562891351E-16, 90.00000000000000000 ) ) ;
#21819=DIRECTION ( 'NONE',  ( -1.350636282998972974E-14, 0.000000000000000000, -1.000000000000000000 ) ) ;
#21832=CARTESIAN_POINT ( 'NONE',  ( -126.6510233831467929, 89.35617925171790432, -28.74099766568598824 ) ) ;
#21834=DIRECTION ( 'NONE',  ( 0.9289202219288174023, 0.3702799228849934510, 6.982962677686266711E-15 ) ) ;
#21845=CARTESIAN_POINT ( 'NONE',  ( -146.0000000000000853, -784.4690652294805204, 30.00000000000641620 ) ) ;
#21864=ORIENTED_EDGE ( 'NONE', *, *, #619, .T. ) ;
#21877=DIRECTION ( 'NONE',  ( -6.982962677686266711E-15, 0.000000000000000000, 1.000000000000000000 ) ) ;
#21878=DIRECTION ( 'NONE',  ( -1.000000000000000000, 1.408839003528726857E-14, 6.982962677686266711E-15 ) ) ;
#21910=CARTESIAN_POINT ( 'NONE',  ( -146.4450000000000500, -784.4690652294805204, 32.50000000000641620 ) ) ;
#21912=AXIS2_PLACEMENT_3D ( 'NONE', #12490, #21834, #14396 ) ;
#21916=CARTESIAN_POINT ( 'NONE',  ( 122.9460700935424171, -1094.388896850127367, -30.32927184981470958 ) ) ;
#21949=LINE ( 'NONE', #12832, #295 ) ;
#21950=CARTESIAN_POINT ( 'NONE',  ( -135.7895026000614678, -1074.740959209980247, 27.50000000000646239 ) ) ;
#21954=CARTESIAN_POINT ( 'NONE',  ( -122.8605704798722087, 82.74225173005940803, -32.05499999999356220 ) ) ;
#21956=CARTESIAN_POINT ( 'NONE',  ( -126.4950807468199798, 89.57684269074619010, -30.66034227022098690 ) ) ;
#21973=STYLED_ITEM('',(#23927),#19781);
#21974=VERTEX_POINT ( 'NONE', #12708 ) ;
#21978=AXIS2_PLACEMENT_3D ( 'NONE', #4385, #22963, #4507 ) ;
#21985=EDGE_CURVE ( 'NONE', #4934, #4706, #21949, .T. ) ;
#21989=CARTESIAN_POINT ( 'NONE',  ( 125.9551925347489316, -1090.334326554368999, -29.66799569545560189 ) ) ;
#22002=EDGE_CURVE ( 'NONE', #3203, #19239, #13833, .T. ) ;
#22003=EDGE_CURVE ( 'NONE', #784, #6379, #5151, .T. ) ;
#22006=ORIENTED_EDGE ( 'NONE', *, *, #12764, .F. ) ;
#22032=LINE ( 'NONE', #16840, #7312 ) ;
#22037=ADVANCED_FACE ( 'NONE', ( #14123 ), #12329, .F. ) ;
#22041=DIRECTION ( 'NONE',  ( 0.6964005597823107463, -0.7176533009294140397, 6.982962677686265922E-15 ) ) ;
#22042=CARTESIAN_POINT ( 'NONE',  ( -155.0000000000000284, -784.4690652294805204, 32.50000000000648015 ) ) ;
#22050=CARTESIAN_POINT ( 'NONE',  ( 171.6502151485109664, 95.33502053007563859, 30.00000000000675726 ) ) ;
#22053=DIRECTION ( 'NONE',  ( -0.9423651898111408132, -0.3345860861306287348, 6.982962677686266711E-15 ) ) ;
#22059=CARTESIAN_POINT ( 'NONE',  ( -146.0000000000000853, -494.4690652294807478, 30.00000000000641620 ) ) ;
#22064=CARTESIAN_POINT ( 'NONE',  ( -136.1024116720894881, -1074.169801158669543, 27.57867027829822604 ) ) ;
#22069=VECTOR ( 'NONE', #14959, 1000.000000000000000 ) ;
#22071=CARTESIAN_POINT ( 'NONE',  ( -126.9537165176728166, 88.92563123478259968, -28.11073331261975028 ) ) ;
#22073=CARTESIAN_POINT ( 'NONE',  ( -194.7500000000004832, -494.4690652294794404, -29.99999999999322498 ) ) ;
#22074=EDGE_LOOP ( 'NONE', ( #8075, #1282, #3588, #658 ) ) ;
#22083=ORIENTED_EDGE ( 'NONE', *, *, #6097, .F. ) ;
#22092=CARTESIAN_POINT ( 'NONE',  ( 125.1337793500214275, -1091.468903702554144, -32.24903484778815255 ) ) ;
#22094=VERTEX_POINT ( 'NONE', #21695 ) ;
#22095=CARTESIAN_POINT ( 'NONE',  ( -122.8605704798723082, 82.74225173005861222, 30.00000000000641620 ) ) ;
#22098=EDGE_CURVE ( 'NONE', #10971, #10033, #10373, .T. ) ;
#22102=CARTESIAN_POINT ( 'NONE',  ( -136.9530201128895328, -1072.586991580760241, -29.34813586885360337 ) ) ;
#22109=CARTESIAN_POINT ( 'NONE',  ( -124.2796999450276587, 81.25594874576239590, 30.00000000000641620 ) ) ;
#22114=ORIENTED_EDGE ( 'NONE', *, *, #1941, .T. ) ;
#22115=CARTESIAN_POINT ( 'NONE',  ( 125.6594390352178152, -1090.745324718712254, 28.47118012353589478 ) ) ;
#22118=CARTESIAN_POINT ( 'NONE',  ( 133.1749347183805696, 79.30613235829001439, 27.57867027829823670 ) ) ;
#22126=EDGE_CURVE ( 'NONE', #4603, #21251, #7231, .T. ) ;
#22127=ADVANCED_FACE ( 'NONE', ( #15920 ), #6728, .F. ) ;
#22131=DIRECTION ( 'NONE',  ( 1.110223024625157172E-14, 0.000000000000000000, -1.000000000000000000 ) ) ;
#22134=CARTESIAN_POINT ( 'NONE',  ( -146.0000000000001137, -784.4690652294805204, 27.94500000000641649 ) ) ;
#22135=DIRECTION ( 'NONE',  ( 0.000000000000000000, 0.000000000000000000, -1.000000000000000000 ) ) ;
#22143=VECTOR ( 'NONE', #12139, 1000.000000000000000 ) ;
#22144=CARTESIAN_POINT ( 'NONE',  ( 126.3653543294818178, 77.28387428943173632, -27.94499999999358053 ) ) ;
#22153=CARTESIAN_POINT ( 'NONE',  ( -146.0000000000005116, -494.4690652294800657, -29.99999999999356604 ) ) ;
#22154=CARTESIAN_POINT ( 'NONE',  ( 126.7787238282401319, 77.44864885511553609, -27.49999999999356248 ) ) ;
#22161=DIRECTION ( 'NONE',  ( -1.350636282998972974E-14, 0.000000000000000000, -1.000000000000000000 ) ) ;
#22168=EDGE_CURVE ( 'NONE', #22922, #8689, #170, .T. ) ;
#22172=AXIS2_PLACEMENT_3D ( 'NONE', #13201, #22314, #2267 ) ;
#22176=VERTEX_POINT ( 'NONE', #22042 ) ;
#22178=CARTESIAN_POINT ( 'NONE',  ( -136.5854636148302461, -1073.276359373527839, 28.11170275877352509 ) ) ;
#22184=CARTESIAN_POINT ( 'NONE',  ( -127.2680799365778199, 88.47518962644144835, -32.24959887471652564 ) ) ;
#22198=DIRECTION ( 'NONE',  ( 1.350636282998972974E-14, 0.000000000000000000, -1.000000000000000000 ) ) ;
#22202=ORIENTED_EDGE ( 'NONE', *, *, #13454, .T. ) ;
#22203=AXIS2_PLACEMENT_3D ( 'NONE', #3164, #5110, #14774 ) ;
#22204=CARTESIAN_POINT ( 'NONE',  ( 153.5653415408403646, -1122.352966361445169, 30.00000000000675726 ) ) ;
#22211=CARTESIAN_POINT ( 'NONE',  ( 125.7666110541939588, -1090.596734011949366, -28.73951976925631513 ) ) ;
#22225=CARTESIAN_POINT ( 'NONE',  ( -134.5482912860055080, -1076.952955187287444, 30.16873261443285870 ) ) ;
#22228=CARTESIAN_POINT ( 'NONE',  ( 155.0000000000000568, -1000.000000000000000, 90.00000000000000000 ) ) ;
#22237=ORIENTED_EDGE ( 'NONE', *, *, #703, .T. ) ;
#22268=VERTEX_POINT ( 'NONE', #2471 ) ;
#22274=FACE_OUTER_BOUND ( 'NONE', #16450, .T. ) ;
#22285=LINE ( 'NONE', #7092, #4588 ) ;
#22288=VERTEX_POINT ( 'NONE', #794 ) ;
#22295=CARTESIAN_POINT ( 'NONE',  ( 126.3653543294811499, 77.28387428943223370, 27.94500000000640227 ) ) ;
#22302=ORIENTED_EDGE ( 'NONE', *, *, #22098, .F. ) ;
#22305=CARTESIAN_POINT ( 'NONE',  ( -155.0000000000000284, -494.4690652294806341, 27.50000000000647660 ) ) ;
#22314=DIRECTION ( 'NONE',  ( 1.000000000000000000, -0.000000000000000000, 6.982962677686266711E-15 ) ) ;
#22320=CARTESIAN_POINT ( 'NONE',  ( -194.7500000000000000, -494.4690652294800657, 32.50000000000675726 ) ) ;
#22337=CIRCLE ( 'NONE', #7673, 2.499999999999998668 ) ;
#22343=DIRECTION ( 'NONE',  ( 0.9289202219288174023, 0.3702799228849934510, 6.982962677686266711E-15 ) ) ;
#22353=CARTESIAN_POINT ( 'NONE',  ( -146.0000000000005400, -204.4690652294800657, -32.05499999999356930 ) ) ;
#22370=CARTESIAN_POINT ( 'NONE',  ( -128.0869692137160598, 87.28547799715779831, 32.48437713430730156 ) ) ;
#22376=FACE_OUTER_BOUND ( 'NONE', #14050, .T. ) ;
#22377=CARTESIAN_POINT ( 'NONE',  ( 119.6158142514527327, -1087.367367941136308, 30.00000000000641620 ) ) ;
#22384=CARTESIAN_POINT ( 'NONE',  ( 131.6538433078038963, 81.80629369879927992, -28.88328940716461801 ) ) ;
#22388=B_SPLINE_CURVE_WITH_KNOTS ( 'NONE', 3,
 ( #18583, #6810, #5812, #25, #14754, #9546, #18475, #5009, #13216, #20516, #5559, #23464, #7376, #3966, #16116, #8751, #21537, #6932, #16907, #2156, #11382, #14203, #14334, #12422, #3174, #10581, #21662, #5120 ),
 .UNSPECIFIED., .F., .F.,
 ( 4, 2, 2, 2, 2, 2, 2, 2, 2, 2, 2, 2, 2, 4 ),
 ( 0.007862850516742125873, 0.008354729399060669900, 0.008846608281379213928, 0.009830366046016345352, 0.01032224492833490673, 0.01081412381065346810, 0.01130600269297203121, 0.01179788157529059259, 0.01278163933992771707, 0.01327351822224628886, 0.01376539710456485890, 0.01425727598688343069, 0.01474915486920200074, 0.01573291263383913216 ),
 .UNSPECIFIED. ) ;
#22392=FACE_OUTER_BOUND ( 'NONE', #2399, .T. ) ;
#22399=CARTESIAN_POINT ( 'NONE',  ( 124.4701338314433201, -1092.369831568443260, -32.49999999999351985 ) ) ;
#22421=DIRECTION ( 'NONE',  ( 0.000000000000000000, 0.000000000000000000, 1.000000000000000000 ) ) ;
#22425=DIRECTION ( 'NONE',  ( 0.000000000000000000, 0.000000000000000000, 1.000000000000000000 ) ) ;
#22457=CYLINDRICAL_SURFACE ( 'NONE', #7029, 2.500000000000002220 ) ;
#22460=DIRECTION ( 'NONE',  ( 0.4924295582441756136, -0.5074575156280946020, -0.7071067811865532349 ) ) ;
#22461=LINE ( 'NONE', #8117, #3717 ) ;
#22479=AXIS2_PLACEMENT_3D ( 'NONE', #9990, #15775, #21203 ) ;
#22496=ORIENTED_EDGE ( 'NONE', *, *, #20882, .T. ) ;
#22503=CARTESIAN_POINT ( 'NONE',  ( 146.4449999999997658, -209.9999999999996874, 30.00000000000641975 ) ) ;
#22505=FACE_BOUND ( 'NONE', #6936, .T. ) ;
#22516=DIRECTION ( 'NONE',  ( -1.000000000000000000, 0.000000000000000000, -6.982962677686266711E-15 ) ) ;
#22522=EDGE_CURVE ( 'NONE', #13741, #17788, #2933, .T. ) ;
#22525=CYLINDRICAL_SURFACE ( 'NONE', #1459, 2.500000000000002220 ) ;
#22543=AXIS2_PLACEMENT_3D ( 'NONE', #17552, #19120, #5971 ) ;
#22546=CIRCLE ( 'NONE', #4823, 2.055000000000001492 ) ;
#22548=ORIENTED_EDGE ( 'NONE', *, *, #288, .T. ) ;
#22556=DIRECTION ( 'NONE',  ( 1.000000000000000000, -0.000000000000000000, 6.982962677686266711E-15 ) ) ;
#22564=ORIENTED_EDGE ( 'NONE', *, *, #13318, .T. ) ;
#22565=EDGE_LOOP ( 'NONE', ( #9455, #22678 ) ) ;
#22569=CIRCLE ( 'NONE', #23356, 2.500000000000002220 ) ;
#22583=CARTESIAN_POINT ( 'NONE',  ( -135.7895026000616667, -1074.740959209979792, -27.49999999999351985 ) ) ;
#22585=ORIENTED_EDGE ( 'NONE', *, *, #14434, .F. ) ;
#22588=AXIS2_PLACEMENT_3D ( 'NONE', #992, #12159, #19579 ) ;
#22593=PLANE ( 'NONE',  #15 ) ;
#22609=VERTEX_POINT ( 'NONE', #5711 ) ;
#22615=CARTESIAN_POINT ( 'NONE',  ( -146.0000000000005400, -204.4690652294800657, -32.05499999999356930 ) ) ;
#22616=ORIENTED_EDGE ( 'NONE', *, *, #3572, .F. ) ;
#22619=VECTOR ( 'NONE', #22556, 1000.000000000000000 ) ;
#22621=CARTESIAN_POINT ( 'NONE',  ( 171.6502151485109948, 95.33502053007563859, 27.50000000000675371 ) ) ;
#22625=FACE_BOUND ( 'NONE', #11993, .T. ) ;
#22630=ORIENTED_EDGE ( 'NONE', *, *, #5297, .T. ) ;
#22631=CARTESIAN_POINT ( 'NONE',  ( 145.0000000000000284, 0.000000000000000000, 90.00000000000000000 ) ) ;
#22644=CARTESIAN_POINT ( 'NONE',  ( -129.6400180686271142, -1072.557589128678273, -32.49999999999356959 ) ) ;
#22650=CARTESIAN_POINT ( 'NONE',  ( -123.1824219776882927, 83.04955713735503764, 27.50000000000641975 ) ) ;
#22659=CONICAL_SURFACE ( 'NONE', #1826, 2.055000000000001492, 0.7853981633974633780 ) ;
#22678=ORIENTED_EDGE ( 'NONE', *, *, #12473, .T. ) ;
#22681=CARTESIAN_POINT ( 'NONE',  ( -126.6049454172962214, 89.42142849840972474, 31.11216498479349468 ) ) ;
#22686=CARTESIAN_POINT ( 'NONE',  ( 146.4449999999998226, -801.0618695410399823, 27.50000000000642331 ) ) ;
#22690=CIRCLE ( 'NONE', #9215, 2.499999999999998668 ) ;
#22691=DIRECTION ( 'NONE',  ( -1.350636282998972974E-14, 0.000000000000000000, -1.000000000000000000 ) ) ;
#22704=ORIENTED_EDGE ( 'NONE', *, *, #22003, .T. ) ;
#22715=CARTESIAN_POINT ( 'NONE',  ( 0.000000000000000000, -1000.000000000000000, 90.00000000000000000 ) ) ;
#22716=LINE ( 'NONE', #7875, #4938 ) ;
#22718=CIRCLE ( 'NONE', #5261, 2.499999999999998668 ) ;
#22720=EDGE_CURVE ( 'NONE', #21618, #3982, #19987, .T. ) ;
#22725=DIRECTION ( 'NONE',  ( -0.7232617928448825673, 0.6905739489807055653, 6.982962677686265922E-15 ) ) ;
#22736=ORIENTED_EDGE ( 'NONE', *, *, #19162, .F. ) ;
#22742=ADVANCED_FACE ( 'NONE', ( #4266, #17186, #21367, #11421, #15029 ), #9586, .T. ) ;
#22748=ADVANCED_FACE ( 'NONE', ( #22376 ), #13872, .F. ) ;
#22753=CARTESIAN_POINT ( 'NONE',  ( 124.2735041650581422, -1092.634345841123377, 27.51597717546058064 ) ) ;
#22777=CARTESIAN_POINT ( 'NONE',  ( -146.0000000000004832, -494.4690652294800657, -27.94499999999356632 ) ) ;
#22794=ORIENTED_EDGE ( 'NONE', *, *, #23057, .F. ) ;
#22796=CARTESIAN_POINT ( 'NONE',  ( -194.7500000000004832, -204.4690652294793836, -29.99999999999322498 ) ) ;
#22801=ORIENTED_EDGE ( 'NONE', *, *, #16705, .F. ) ;
#22803=DIRECTION ( 'NONE',  ( 0.000000000000000000, 0.000000000000000000, -1.000000000000000000 ) ) ;
#22831=VERTEX_POINT ( 'NONE', #16193 ) ;
#22834=ADVANCED_FACE ( 'NONE', ( #7114 ), #1672, .T. ) ;
#22835=EDGE_LOOP ( 'NONE', ( #6184, #14761 ) ) ;
#22876=EDGE_CURVE ( 'NONE', #11798, #10962, #15774, .T. ) ;
#22899=DIRECTION ( 'NONE',  ( -1.110223024625155594E-14, 0.000000000000000000, -1.000000000000000000 ) ) ;
#22900=LINE ( 'NONE', #4444, #20380 ) ;
#22914=CARTESIAN_POINT ( 'NONE',  ( -127.8094121079452776, 87.69139705313205013, 32.50000000000647304 ) ) ;
#22916=VERTEX_POINT ( 'NONE', #4951 ) ;
#22920=CARTESIAN_POINT ( 'NONE',  ( -145.0000000000000284, -1000.000000000000000, 90.00000000000000000 ) ) ;
#22922=VERTEX_POINT ( 'NONE', #14611 ) ;
#22934=ORIENTED_EDGE ( 'NONE', *, *, #1512, .T. ) ;
#22946=CARTESIAN_POINT ( 'NONE',  ( 146.0000000000001990, -801.0618695410406644, -27.94499999999356632 ) ) ;
#22954=EDGE_CURVE ( 'NONE', #846, #8260, #19585, .T. ) ;
#22958=FILL_AREA_STYLE ('',( #6072 ) ) ;
#22963=DIRECTION ( 'NONE',  ( 1.000000000000000000, -1.408839003528726857E-14, -6.982962677686266711E-15 ) ) ;
#22992=DIRECTION ( 'NONE',  ( -1.000000000000000000, 0.000000000000000000, -6.982962677686266711E-15 ) ) ;
#22994=ORIENTED_EDGE ( 'NONE', *, *, #6902, .F. ) ;
#22998=DIRECTION ( 'NONE',  ( 1.110223024625157172E-14, 0.000000000000000000, -1.000000000000000000 ) ) ;
#23010=CARTESIAN_POINT ( 'NONE',  ( -155.0000000000000284, -784.4690652294798383, -29.99999999999350564 ) ) ;
#23020=ORIENTED_EDGE ( 'NONE', *, *, #15687, .T. ) ;
#23024=ORIENTED_EDGE ( 'NONE', *, *, #1946, .F. ) ;
#23031=CARTESIAN_POINT ( 'NONE',  ( -127.0272233253972587, 88.82062435171954462, 31.99235058689528444 ) ) ;
#23035=CARTESIAN_POINT ( 'NONE',  ( -135.4738523116357953, -1075.311763300249822, -27.57873596473009314 ) ) ;
#23044=VERTEX_POINT ( 'NONE', #2390 ) ;
#23057=EDGE_CURVE ( 'NONE', #21068, #885, #22900, .T. ) ;
#23067=VECTOR ( 'NONE', #1993, 1000.000000000000000 ) ;
#23080=CARTESIAN_POINT ( 'NONE',  ( -175.1609685624542578, -1088.719770019218458, -29.99999999999322498 ) ) ;
#23091=AXIS2_PLACEMENT_3D ( 'NONE', #5056, #19761, #2229 ) ;
#23097=EDGE_LOOP ( 'NONE', ( #11689, #17105 ) ) ;
#23119=DIRECTION ( 'NONE',  ( -4.862939117679700002E-15, 5.011346215908450209E-15, 1.000000000000000000 ) ) ;
#23124=CARTESIAN_POINT ( 'NONE',  ( 145.0000000000000284, -500.0000000000000000, 27.50000000000001066 ) ) ;
#23136=CARTESIAN_POINT ( 'NONE',  ( 131.5594662024482489, 81.95796442704008200, 30.65375098132849985 ) ) ;
#23139=DIRECTION ( 'NONE',  ( 0.9289202219288174023, 0.3702799228849934510, 6.982962677686266711E-15 ) ) ;
#23140=VERTEX_POINT ( 'NONE', #17128 ) ;
#23144=EDGE_CURVE ( 'NONE', #8155, #12774, #21170, .T. ) ;
#23145=LINE ( 'NONE', #17246, #16369 ) ;
#23148=CARTESIAN_POINT ( 'NONE',  ( -129.2206655591605511, -1072.408698320350595, 32.05500000000640171 ) ) ;
#23159=ORIENTED_EDGE ( 'NONE', *, *, #12004, .F. ) ;
#23167=CARTESIAN_POINT ( 'NONE',  ( -126.4950807468203919, 89.57684269074565009, 29.33965772977898823 ) ) ;
#23170=ORIENTED_EDGE ( 'NONE', *, *, #2196, .T. ) ;
#23177=ADVANCED_FACE ( 'NONE', ( #18927 ), #17593, .F. ) ;
#23180=EDGE_CURVE ( 'NONE', #15388, #18827, #11979, .T. ) ;
#23185=LINE ( 'NONE', #6764, #19532 ) ;
#23188=ORIENTED_EDGE ( 'NONE', *, *, #10132, .F. ) ;
#23198=EDGE_LOOP ( 'NONE', ( #11666, #7832, #23518, #14885 ) ) ;
#23201=DIRECTION ( 'NONE',  ( -0.9423651898111408132, -0.3345860861306287348, 6.982962677686266711E-15 ) ) ;
#23203=ORIENTED_EDGE ( 'NONE', *, *, #10568, .F. ) ;
#23209=EDGE_CURVE ( 'NONE', #3131, #15388, #14263, .T. ) ;
#23216=ORIENTED_EDGE ( 'NONE', *, *, #23711, .F. ) ;
#23228=CARTESIAN_POINT ( 'NONE',  ( -194.7500000000005116, -784.4690652294792699, -32.49999999999322853 ) ) ;
#23254=CIRCLE ( 'NONE', #20544, 2.500000000000002220 ) ;
#23267=ORIENTED_EDGE ( 'NONE', *, *, #3710, .T. ) ;
#23280=CARTESIAN_POINT ( 'NONE',  ( -146.0000000000005116, -204.4690652294800657, -29.99999999999356604 ) ) ;
#23281=ADVANCED_FACE ( 'NONE', ( #10872, #21458, #6980 ), #14013, .T. ) ;
#23282=ORIENTED_EDGE ( 'NONE', *, *, #21677, .F. ) ;
#23287=CARTESIAN_POINT ( 'NONE',  ( 134.1180124237195912, 77.70044921554776352, -29.67081494451416646 ) ) ;
#23294=DIRECTION ( 'NONE',  ( -0.7232617928448825673, 0.6905739489807055653, 6.982962677686266711E-15 ) ) ;
#23302=CIRCLE ( 'NONE', #12946, 2.499999999999998668 ) ;
#23310=CARTESIAN_POINT ( 'NONE',  ( -136.3242110351073109, -1073.761323382753744, 32.24990070396070507 ) ) ;
#23311=DIRECTION ( 'NONE',  ( -1.000000000000000000, 1.408839003528726857E-14, 6.982962677686266711E-15 ) ) ;
#23315=DIRECTION ( 'NONE',  ( -1.110223024625157172E-14, 0.000000000000000000, -1.000000000000000000 ) ) ;
#23319=CARTESIAN_POINT ( 'NONE',  ( 124.6651547408753800, -1092.106598813447590, -27.51562286569270199 ) ) ;
#23334=CONICAL_SURFACE ( 'NONE', #22172, 2.055000000000001492, 0.7853981633974633780 ) ;
#23336=FACE_OUTER_BOUND ( 'NONE', #20171, .T. ) ;
#23342=CIRCLE ( 'NONE', #5219, 2.500000000000002220 ) ;
#23346=CARTESIAN_POINT ( 'NONE',  ( -129.6400180686265173, -1072.557589128678728, 30.00000000000641975 ) ) ;
#23348=ADVANCED_FACE ( 'NONE', ( #17843 ), #14249, .F. ) ;
#23355=CARTESIAN_POINT ( 'NONE',  ( 121.0905917848626814, -1085.936264790783525, 30.00000000000641620 ) ) ;
#23356=AXIS2_PLACEMENT_3D ( 'NONE', #23508, #16270, #7072 ) ;
#23372=CARTESIAN_POINT ( 'NONE',  ( 132.8404720734530144, 79.86494211668951948, 32.50000000000646594 ) ) ;
#23379=EDGE_CURVE ( 'NONE', #4603, #22094, #9502, .T. ) ;
#23387=CARTESIAN_POINT ( 'NONE',  ( -146.4450000000000784, -494.4690652294807478, 30.00000000000641975 ) ) ;
#23391=ORIENTED_EDGE ( 'NONE', *, *, #6658, .F. ) ;
#23398=DIRECTION ( 'NONE',  ( -1.000000000000000000, 1.408839003528726857E-14, 6.982962677686266711E-15 ) ) ;
#23404=CARTESIAN_POINT ( 'NONE',  ( -134.8618744214602714, -1076.402150461712608, -28.33934113061011217 ) ) ;
#23408=FACE_OUTER_BOUND ( 'NONE', #19691, .T. ) ;
#23424=CARTESIAN_POINT ( 'NONE',  ( -123.1824219776881790, 83.04955713735581924, -32.49999999999356959 ) ) ;
#23432=VECTOR ( 'NONE', #15373, 1000.000000000000000 ) ;
#23441=DIRECTION ( 'NONE',  ( -6.753181414994864868E-15, 6.753181414994864868E-15, -1.000000000000000000 ) ) ;
#23451=CYLINDRICAL_SURFACE ( 'NONE', #22203, 2.500000000000002220 ) ;
#23457=FACE_OUTER_BOUND ( 'NONE', #9648, .T. ) ;
#23463=ORIENTED_EDGE ( 'NONE', *, *, #13098, .T. ) ;
#23464=CARTESIAN_POINT ( 'NONE',  ( -129.2447185937758718, 85.56171376302411602, -29.18615827854497624 ) ) ;
#23468=CARTESIAN_POINT ( 'NONE',  ( 133.6263423143003877, 78.54310546248494518, 31.99235058689527733 ) ) ;
#23475=CARTESIAN_POINT ( 'NONE',  ( -129.2206655591605511, -1072.408698320350595, 32.05500000000641592 ) ) ;
#23480=DIRECTION ( 'NONE',  ( 0.000000000000000000, 0.000000000000000000, -1.000000000000000000 ) ) ;
#23487=AXIS2_PLACEMENT_3D ( 'NONE', #16266, #8776, #21445 ) ;
#23494=CARTESIAN_POINT ( 'NONE',  ( -146.4450000000001069, -204.4690652294807194, 27.50000000000642331 ) ) ;
#23495=AXIS2_PLACEMENT_3D ( 'NONE', #3993, #13237, #20430 ) ;
#23500=LINE ( 'NONE', #7067, #6903 ) ;
#23508=CARTESIAN_POINT ( 'NONE',  ( 145.0000000000000284, -500.0000000000000000, 30.00000000000001421 ) ) ;
#23511=FACE_OUTER_BOUND ( 'NONE', #18768, .T. ) ;
#23512=DIRECTION ( 'NONE',  ( 1.000000000000000000, 0.000000000000000000, 0.000000000000000000 ) ) ;
#23518=ORIENTED_EDGE ( 'NONE', *, *, #19334, .F. ) ;
#23528=CARTESIAN_POINT ( 'NONE',  ( 0.000000000000000000, 0.000000000000000000, 90.00000000000000000 ) ) ;
#23529=CARTESIAN_POINT ( 'NONE',  ( -155.0000000000000284, -1000.000000000000000, 90.00000000000000000 ) ) ;
#23542=CYLINDRICAL_SURFACE ( 'NONE', #9033, 2.500000000000002220 ) ;
#23546=DIRECTION ( 'NONE',  ( -1.000000000000000000, 1.408839003528726857E-14, 6.982962677686266711E-15 ) ) ;
#23552=ORIENTED_EDGE ( 'NONE', *, *, #23379, .T. ) ;
#23570=LINE ( 'NONE', #1591, #15347 ) ;
#23576=DIRECTION ( 'NONE',  ( 1.000000000000000000, -0.000000000000000000, 6.982962677686266711E-15 ) ) ;
#23578=EDGE_LOOP ( 'NONE', ( #17588, #18552 ) ) ;
#23594=CARTESIAN_POINT ( 'NONE',  ( 133.2563391751588142, 79.16925799295282218, 32.37408494914630097 ) ) ;
#23596=LINE ( 'NONE', #7050, #19825 ) ;
#23618=ORIENTED_EDGE ( 'NONE', *, *, #1633, .T. ) ;
#23620=ADVANCED_FACE ( 'NONE', ( #13751 ), #13643, .F. ) ;
#23633=CARTESIAN_POINT ( 'NONE',  ( -129.2206655591611764, -1072.408698320350140, -29.99999999999356604 ) ) ;
#23634=CARTESIAN_POINT ( 'NONE',  ( -146.0000000000000853, -784.4690652294805204, 30.00000000000641620 ) ) ;
#23635=ORIENTED_EDGE ( 'NONE', *, *, #9886, .F. ) ;
#23641=CIRCLE ( 'NONE', #7838, 2.500000000000002220 ) ;
#23646=CARTESIAN_POINT ( 'NONE',  ( -129.6400180686264605, -1072.557589128678728, 32.50000000000641620 ) ) ;
#23651=CARTESIAN_POINT ( 'NONE',  ( -126.6511612778951132, 89.35598455390456252, -31.25955389945143281 ) ) ;
#23653=EDGE_CURVE ( 'NONE', #1928, #21308, #17458, .T. ) ;
#23655=FACE_OUTER_BOUND ( 'NONE', #20992, .T. ) ;
#23660=FACE_OUTER_BOUND ( 'NONE', #5220, .T. ) ;
#23661=CARTESIAN_POINT ( 'NONE',  ( 0.000000000000000000, -1000.000000000000000, -90.00000000000000000 ) ) ;
#23664=AXIS2_PLACEMENT_3D ( 'NONE', #9320, #7600, #5674 ) ;
#23673=CARTESIAN_POINT ( 'NONE',  ( 125.8137507114119558, -1090.531233726929941, -31.11299551804367880 ) ) ;
#23690=CARTESIAN_POINT ( 'NONE',  ( 145.9999999999998295, -801.0618695410399823, 27.94500000000641649 ) ) ;
#23691=CARTESIAN_POINT ( 'NONE',  ( 119.6158142514525622, -1087.367367941136990, -29.99999999999356604 ) ) ;
#23711=EDGE_CURVE ( 'NONE', #6064, #16055, #10426, .T. ) ;
#23714=AXIS2_PLACEMENT_3D ( 'NONE', #22059, #5523, #16403 ) ;
#23725=CARTESIAN_POINT ( 'NONE',  ( -155.0000000000000284, -494.4690652294799520, -32.49999999999350564 ) ) ;
#23729=CARTESIAN_POINT ( 'NONE',  ( 123.8014913250395921, -1093.264216588539966, -32.24959887471653985 ) ) ;
#23745=DIRECTION ( 'NONE',  ( -1.000000000000000000, 1.408839003528726857E-14, 6.982962677686266711E-15 ) ) ;
#23755=EDGE_LOOP ( 'NONE', ( #21091, #2485 ) ) ;
#23768=ADVANCED_FACE ( 'NONE', ( #5248 ), #21194, .F. ) ;
#23921=COLOUR_RGB('Black',0.12,0.14,0.17);
#23922=FILL_AREA_STYLE_COLOUR('',#23921);
#23923=FILL_AREA_STYLE('',(#23922));
#23924=SURFACE_STYLE_FILL_AREA(#23923);
#23925=SURFACE_SIDE_STYLE('',(#23924));
#23926=SURFACE_STYLE_USAGE(.BOTH.,#23925);
#23927=PRESENTATION_STYLE_ASSIGNMENT((#23926));
ENDSEC;
END-ISO-10303-21;
